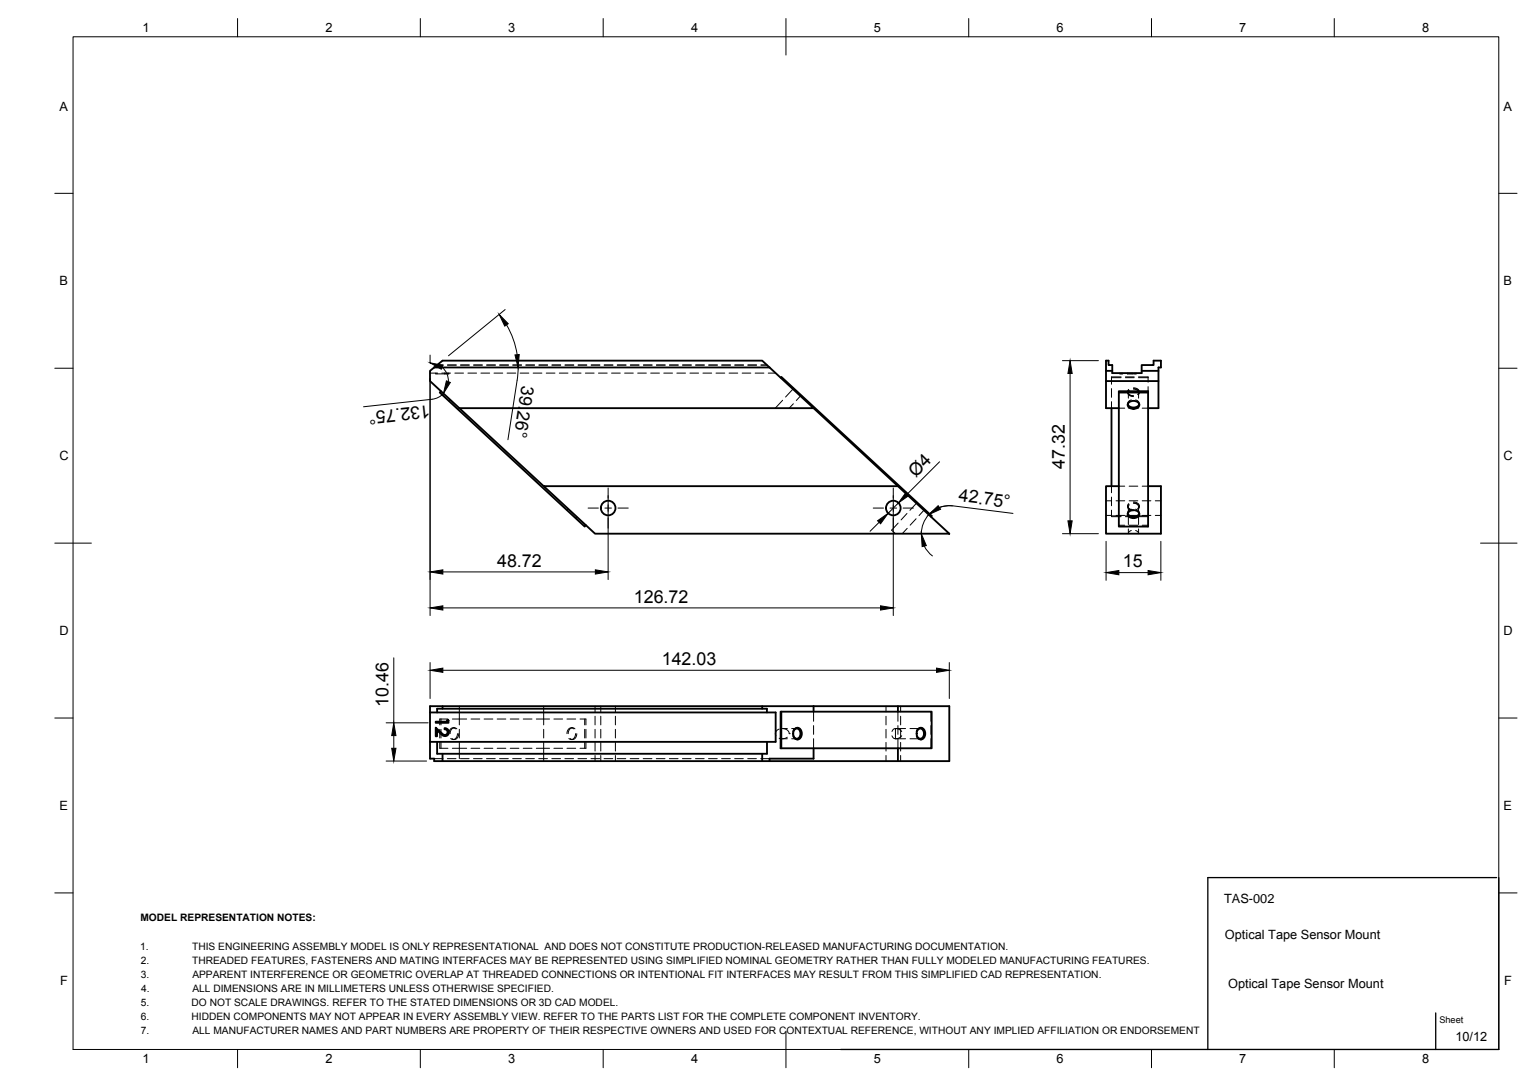
ISO-10303-21;
HEADER;
/* Generated by software containing ST-Developer
 * from STEP Tools, Inc. (www.steptools.com) 
 */

FILE_DESCRIPTION(
/* description */ ('STEP AP214'),
/* implementation_level */ '2;1');

FILE_NAME(
/* name */ 'Optical Tape Sensor Mount.step',
/* time_stamp */ '2026-11-04T19:38:14-08:00',
/* author */ (''),
/* organization */ (''),
/* preprocessor_version */ 'ST-DEVELOPER v20.2',
/* originating_system */ 'Autodesk Translation Framework v15.17.0.0',
/* authorisation */ '');

FILE_SCHEMA (('AUTOMOTIVE_DESIGN { 1 0 10303 214 3 1 1 }'));
ENDSEC;

DATA;
#10=MECHANICAL_DESIGN_GEOMETRIC_PRESENTATION_REPRESENTATION('',(#477),#36668);
#53=B_SPLINE_SURFACE_WITH_KNOTS('',3,1,((#33152,#33153),(#33154,#33155),
(#33156,#33157),(#33158,#33159),(#33160,#33161),(#33162,#33163),(#33164,
#33165),(#33166,#33167),(#33168,#33169),(#33170,#33171),(#33172,#33173),
(#33174,#33175),(#33176,#33177),(#33178,#33179),(#33180,#33181),(#33182,
#33183),(#33184,#33185),(#33186,#33187),(#33188,#33189)),.UNSPECIFIED.,
 .F.,.F.,.F.,(4,1,1,1,1,1,1,1,1,1,1,1,1,1,1,1,4),(2,2),(0.,0.0619654006870562,
0.122121905638296,0.180988496849837,0.239933216451894,0.299905831106524,
0.359988847476984,0.421775741741642,0.486575826421121,0.551534804619736,
0.615017542759975,0.677258616661654,0.739729962362713,0.803050102662949,
0.866495132015699,0.931973474177149,1.),(0.,0.0239999999999995),
 .UNSPECIFIED.);
#54=B_SPLINE_SURFACE_WITH_KNOTS('',3,1,((#33213,#33214),(#33215,#33216),
(#33217,#33218),(#33219,#33220),(#33221,#33222),(#33223,#33224),(#33225,
#33226),(#33227,#33228),(#33229,#33230),(#33231,#33232),(#33233,#33234),
(#33235,#33236),(#33237,#33238),(#33239,#33240),(#33241,#33242)),
 .UNSPECIFIED.,.F.,.F.,.F.,(4,1,1,1,1,1,1,1,1,1,1,1,4),(2,2),(0.,0.110802643801324,
0.212829202347773,0.306101309823115,0.390647321116006,0.46692446936085,
0.534481039284033,0.593586940965671,0.644557004508714,0.736200452629367,
0.825024025618864,0.911985584829753,1.),(0.,0.0239999999999995),
 .UNSPECIFIED.);
#55=B_SPLINE_SURFACE_WITH_KNOTS('',3,1,((#33280,#33281),(#33282,#33283),
(#33284,#33285),(#33286,#33287),(#33288,#33289),(#33290,#33291),(#33292,
#33293),(#33294,#33295),(#33296,#33297),(#33298,#33299),(#33300,#33301),
(#33302,#33303),(#33304,#33305),(#33306,#33307),(#33308,#33309)),
 .UNSPECIFIED.,.F.,.F.,.F.,(4,1,1,1,1,1,1,1,1,1,1,1,4),(2,2),(0.,0.0987013748863702,
0.195670680385855,0.292419992908961,0.391339286967469,0.444458741764931,
0.504224579154748,0.570347591406357,0.642913825979479,0.722289816523959,
0.807922721202247,0.900470366297794,1.),(0.,0.0239999999999995),
 .UNSPECIFIED.);
#56=B_SPLINE_SURFACE_WITH_KNOTS('',3,1,((#33327,#33328),(#33329,#33330),
(#33331,#33332),(#33333,#33334),(#33335,#33336),(#33337,#33338),(#33339,
#33340),(#33341,#33342),(#33343,#33344),(#33345,#33346),(#33347,#33348),
(#33349,#33350),(#33351,#33352),(#33353,#33354),(#33355,#33356),(#33357,
#33358),(#33359,#33360),(#33361,#33362),(#33363,#33364)),.UNSPECIFIED.,
 .F.,.F.,.F.,(4,1,1,1,1,1,1,1,1,1,1,1,1,1,1,1,4),(2,2),(0.,0.0694796363669832,
0.136525003539142,0.200800892873422,0.263983206913328,0.325711144761188,
0.38727051407573,0.449492780531563,0.51295519576285,0.576266397070109,0.637574966831173,
0.697901098424494,0.757558279411561,0.81658750436506,0.876645756608308,
0.937285872938128,1.),(0.,0.0240000000000054),.UNSPECIFIED.);
#57=B_SPLINE_SURFACE_WITH_KNOTS('',3,1,((#33386,#33387),(#33388,#33389),
(#33390,#33391),(#33392,#33393),(#33394,#33395),(#33396,#33397),(#33398,
#33399),(#33400,#33401),(#33402,#33403),(#33404,#33405),(#33406,#33407),
(#33408,#33409),(#33410,#33411),(#33412,#33413),(#33414,#33415),(#33416,
#33417),(#33418,#33419),(#33420,#33421),(#33422,#33423)),.UNSPECIFIED.,
 .F.,.F.,.F.,(4,1,1,1,1,1,1,1,1,1,1,1,1,1,1,1,4),(2,2),(0.,0.0687907943906199,
0.135103289431132,0.198978674310652,0.261904299780862,0.323494969367974,
0.385195377966055,0.446969238740777,0.509764776703136,0.572250568847369,
0.633405175661155,0.693251162921754,0.752583162785671,0.812579266153423,
0.873275084920192,0.93554994289503,1.),(0.,0.0239999999999995),
 .UNSPECIFIED.);
#58=B_SPLINE_SURFACE_WITH_KNOTS('',3,1,((#33449,#33450),(#33451,#33452),
(#33453,#33454),(#33455,#33456),(#33457,#33458),(#33459,#33460),(#33461,
#33462),(#33463,#33464),(#33465,#33466),(#33467,#33468),(#33469,#33470),
(#33471,#33472),(#33473,#33474),(#33475,#33476),(#33477,#33478),(#33479,
#33480),(#33481,#33482),(#33483,#33484),(#33485,#33486)),.UNSPECIFIED.,
 .F.,.F.,.F.,(4,1,1,1,1,1,1,1,1,1,1,1,1,1,1,1,4),(2,2),(0.,0.064429890715421,
0.126529667073554,0.186743666835525,0.245897683478137,0.304053106820992,
0.362195516217047,0.420654638852463,0.480330856318868,0.540662876085596,
0.600743511343268,0.661981856833518,0.724480055372708,0.789067141037209,
0.856333336778513,0.926362064011592,1.),(0.,0.0239999999999995),
 .UNSPECIFIED.);
#345=B_SPLINE_CURVE_WITH_KNOTS('',3,(#33030,#33031,#33032,#33033,#33034,
#33035,#33036,#33037,#33038,#33039,#33040,#33041,#33042,#33043,#33044,#33045,
#33046,#33047,#33048),.UNSPECIFIED.,.F.,.F.,(4,1,1,1,1,1,1,1,1,1,1,1,1,
1,1,1,4),(0.,0.064429890715421,0.126529667073554,0.186743666835525,0.245897683478137,
0.304053106820992,0.362195516217047,0.420654638852463,0.480330856318868,
0.540662876085596,0.600743511343268,0.661981856833518,0.724480055372708,
0.789067141037209,0.856333336778513,0.926362064011592,1.),.UNSPECIFIED.);
#346=B_SPLINE_CURVE_WITH_KNOTS('',3,(#33050,#33051,#33052,#33053,#33054,
#33055,#33056,#33057,#33058,#33059,#33060,#33061,#33062,#33063,#33064,#33065,
#33066,#33067,#33068),.UNSPECIFIED.,.F.,.F.,(4,1,1,1,1,1,1,1,1,1,1,1,1,
1,1,1,4),(0.,0.0619654006870562,0.122121905638296,0.180988496849837,0.239933216451894,
0.299905831106524,0.359988847476984,0.421775741741642,0.486575826421121,
0.551534804619736,0.615017542759975,0.677258616661654,0.739729962362713,
0.803050102662949,0.866495132015699,0.931973474177149,1.),.UNSPECIFIED.);
#347=B_SPLINE_CURVE_WITH_KNOTS('',3,(#33070,#33071,#33072,#33073,#33074,
#33075,#33076,#33077,#33078,#33079,#33080,#33081,#33082,#33083,#33084),
 .UNSPECIFIED.,.F.,.F.,(4,1,1,1,1,1,1,1,1,1,1,1,4),(0.,0.110802643801324,
0.212829202347773,0.306101309823115,0.390647321116006,0.46692446936085,
0.534481039284033,0.593586940965671,0.644557004508714,0.736200452629367,
0.825024025618864,0.911985584829753,1.),.UNSPECIFIED.);
#348=B_SPLINE_CURVE_WITH_KNOTS('',3,(#33096,#33097,#33098,#33099,#33100,
#33101,#33102,#33103,#33104,#33105,#33106,#33107,#33108,#33109,#33110),
 .UNSPECIFIED.,.F.,.F.,(4,1,1,1,1,1,1,1,1,1,1,1,4),(0.,0.0987013748863702,
0.195670680385855,0.292419992908961,0.391339286967469,0.444458741764931,
0.504224579154748,0.570347591406357,0.642913825979479,0.722289816523959,
0.807922721202247,0.900470366297794,1.),.UNSPECIFIED.);
#349=B_SPLINE_CURVE_WITH_KNOTS('',3,(#33112,#33113,#33114,#33115,#33116,
#33117,#33118,#33119,#33120,#33121,#33122,#33123,#33124,#33125,#33126,#33127,
#33128,#33129,#33130),.UNSPECIFIED.,.F.,.F.,(4,1,1,1,1,1,1,1,1,1,1,1,1,
1,1,1,4),(0.,0.0694796363669832,0.136525003539142,0.200800892873422,0.263983206913328,
0.325711144761188,0.38727051407573,0.449492780531563,0.51295519576285,0.576266397070109,
0.637574966831173,0.697901098424494,0.757558279411561,0.81658750436506,
0.876645756608308,0.937285872938128,1.),.UNSPECIFIED.);
#350=B_SPLINE_CURVE_WITH_KNOTS('',3,(#33132,#33133,#33134,#33135,#33136,
#33137,#33138,#33139,#33140,#33141,#33142,#33143,#33144,#33145,#33146,#33147,
#33148,#33149,#33150),.UNSPECIFIED.,.F.,.F.,(4,1,1,1,1,1,1,1,1,1,1,1,1,
1,1,1,4),(0.,0.0687907943906199,0.135103289431132,0.198978674310652,0.261904299780862,
0.323494969367974,0.385195377966055,0.446969238740777,0.509764776703136,
0.572250568847369,0.633405175661155,0.693251162921754,0.752583162785671,
0.812579266153423,0.873275084920192,0.93554994289503,1.),.UNSPECIFIED.);
#351=B_SPLINE_CURVE_WITH_KNOTS('',3,(#33192,#33193,#33194,#33195,#33196,
#33197,#33198,#33199,#33200,#33201,#33202,#33203,#33204,#33205,#33206,#33207,
#33208,#33209,#33210),.UNSPECIFIED.,.F.,.F.,(4,1,1,1,1,1,1,1,1,1,1,1,1,
1,1,1,4),(0.,0.0619654006870562,0.122121905638296,0.180988496849837,0.239933216451894,
0.299905831106524,0.359988847476984,0.421775741741642,0.486575826421121,
0.551534804619736,0.615017542759975,0.677258616661654,0.739729962362713,
0.803050102662949,0.866495132015699,0.931973474177149,1.),.UNSPECIFIED.);
#352=B_SPLINE_CURVE_WITH_KNOTS('',3,(#33244,#33245,#33246,#33247,#33248,
#33249,#33250,#33251,#33252,#33253,#33254,#33255,#33256,#33257,#33258),
 .UNSPECIFIED.,.F.,.F.,(4,1,1,1,1,1,1,1,1,1,1,1,4),(0.,0.110802643801324,
0.212829202347773,0.306101309823115,0.390647321116006,0.46692446936085,
0.534481039284033,0.593586940965671,0.644557004508714,0.736200452629367,
0.825024025618864,0.911985584829753,1.),.UNSPECIFIED.);
#353=B_SPLINE_CURVE_WITH_KNOTS('',3,(#33311,#33312,#33313,#33314,#33315,
#33316,#33317,#33318,#33319,#33320,#33321,#33322,#33323,#33324,#33325),
 .UNSPECIFIED.,.F.,.F.,(4,1,1,1,1,1,1,1,1,1,1,1,4),(0.,0.0987013748863702,
0.195670680385855,0.292419992908961,0.391339286967469,0.444458741764931,
0.504224579154748,0.570347591406357,0.642913825979479,0.722289816523959,
0.807922721202247,0.900470366297794,1.),.UNSPECIFIED.);
#354=B_SPLINE_CURVE_WITH_KNOTS('',3,(#33366,#33367,#33368,#33369,#33370,
#33371,#33372,#33373,#33374,#33375,#33376,#33377,#33378,#33379,#33380,#33381,
#33382,#33383,#33384),.UNSPECIFIED.,.F.,.F.,(4,1,1,1,1,1,1,1,1,1,1,1,1,
1,1,1,4),(0.,0.0694796363669832,0.136525003539142,0.200800892873422,0.263983206913328,
0.325711144761188,0.38727051407573,0.449492780531563,0.51295519576285,0.576266397070109,
0.637574966831173,0.697901098424494,0.757558279411561,0.81658750436506,
0.876645756608308,0.937285872938128,1.),.UNSPECIFIED.);
#355=B_SPLINE_CURVE_WITH_KNOTS('',3,(#33425,#33426,#33427,#33428,#33429,
#33430,#33431,#33432,#33433,#33434,#33435,#33436,#33437,#33438,#33439,#33440,
#33441,#33442,#33443),.UNSPECIFIED.,.F.,.F.,(4,1,1,1,1,1,1,1,1,1,1,1,1,
1,1,1,4),(0.,0.0687907943906199,0.135103289431132,0.198978674310652,0.261904299780862,
0.323494969367974,0.385195377966055,0.446969238740777,0.509764776703136,
0.572250568847369,0.633405175661155,0.693251162921754,0.752583162785671,
0.812579266153423,0.873275084920192,0.93554994289503,1.),.UNSPECIFIED.);
#356=B_SPLINE_CURVE_WITH_KNOTS('',3,(#33487,#33488,#33489,#33490,#33491,
#33492,#33493,#33494,#33495,#33496,#33497,#33498,#33499,#33500,#33501,#33502,
#33503,#33504,#33505),.UNSPECIFIED.,.F.,.F.,(4,1,1,1,1,1,1,1,1,1,1,1,1,
1,1,1,4),(0.,0.064429890715421,0.126529667073554,0.186743666835525,0.245897683478137,
0.304053106820992,0.362195516217047,0.420654638852463,0.480330856318868,
0.540662876085596,0.600743511343268,0.661981856833518,0.724480055372708,
0.789067141037209,0.856333336778513,0.926362064011592,1.),.UNSPECIFIED.);
#430=ELLIPSE('',#19087,1.9066404831829,1.40000000000002);
#431=ELLIPSE('',#19093,1.9066404831826,1.40000000000005);
#457=SHAPE_REPRESENTATION_RELATIONSHIP('SRR','None',#36713,#467);
#467=ADVANCED_BREP_SHAPE_REPRESENTATION('',(#487),#36665);
#477=STYLED_ITEM('',(#36769),#487);
#487=MANIFOLD_SOLID_BREP('Body1',#17800);
#702=CYLINDRICAL_SURFACE('',#19086,1.4);
#703=CYLINDRICAL_SURFACE('',#19092,1.4);
#704=CYLINDRICAL_SURFACE('',#19121,1.6);
#705=CYLINDRICAL_SURFACE('',#19123,1.6);
#706=CYLINDRICAL_SURFACE('',#19138,2.);
#707=CYLINDRICAL_SURFACE('',#19139,2.);
#708=CYLINDRICAL_SURFACE('',#19147,1.6);
#709=CYLINDRICAL_SURFACE('',#19149,1.6);
#942=FACE_BOUND('',#3354,.T.);
#943=FACE_BOUND('',#3355,.T.);
#944=FACE_BOUND('',#3358,.T.);
#945=FACE_BOUND('',#3359,.T.);
#946=FACE_BOUND('',#3361,.T.);
#947=FACE_BOUND('',#3362,.T.);
#948=FACE_BOUND('',#3367,.T.);
#949=FACE_BOUND('',#3371,.T.);
#950=FACE_BOUND('',#3373,.T.);
#951=FACE_BOUND('',#3381,.T.);
#952=FACE_BOUND('',#3382,.T.);
#953=FACE_BOUND('',#3387,.T.);
#954=FACE_BOUND('',#3396,.T.);
#955=FACE_BOUND('',#3397,.T.);
#1440=CIRCLE('',#19088,1.4);
#1441=CIRCLE('',#19090,1.4);
#1442=CIRCLE('',#19091,1.4);
#1443=CIRCLE('',#19094,1.4);
#1444=CIRCLE('',#19118,1.6);
#1445=CIRCLE('',#19120,1.6);
#1446=CIRCLE('',#19122,1.6);
#1447=CIRCLE('',#19124,1.6);
#1448=CIRCLE('',#19132,2.);
#1449=CIRCLE('',#19133,2.);
#1450=CIRCLE('',#19135,2.);
#1451=CIRCLE('',#19136,2.);
#1452=CIRCLE('',#19144,1.6);
#1453=CIRCLE('',#19146,1.6);
#1454=CIRCLE('',#19148,1.6);
#1455=CIRCLE('',#19150,1.6);
#2217=FACE_OUTER_BOUND('',#3314,.T.);
#2218=FACE_OUTER_BOUND('',#3315,.T.);
#2219=FACE_OUTER_BOUND('',#3316,.T.);
#2220=FACE_OUTER_BOUND('',#3317,.T.);
#2221=FACE_OUTER_BOUND('',#3318,.T.);
#2222=FACE_OUTER_BOUND('',#3319,.T.);
#2223=FACE_OUTER_BOUND('',#3320,.T.);
#2224=FACE_OUTER_BOUND('',#3321,.T.);
#2225=FACE_OUTER_BOUND('',#3322,.T.);
#2226=FACE_OUTER_BOUND('',#3323,.T.);
#2227=FACE_OUTER_BOUND('',#3324,.T.);
#2228=FACE_OUTER_BOUND('',#3325,.T.);
#2229=FACE_OUTER_BOUND('',#3326,.T.);
#2230=FACE_OUTER_BOUND('',#3327,.T.);
#2231=FACE_OUTER_BOUND('',#3328,.T.);
#2232=FACE_OUTER_BOUND('',#3329,.T.);
#2233=FACE_OUTER_BOUND('',#3330,.T.);
#2234=FACE_OUTER_BOUND('',#3331,.T.);
#2235=FACE_OUTER_BOUND('',#3332,.T.);
#2236=FACE_OUTER_BOUND('',#3333,.T.);
#2237=FACE_OUTER_BOUND('',#3334,.T.);
#2238=FACE_OUTER_BOUND('',#3335,.T.);
#2239=FACE_OUTER_BOUND('',#3336,.T.);
#2240=FACE_OUTER_BOUND('',#3337,.T.);
#2241=FACE_OUTER_BOUND('',#3338,.T.);
#2242=FACE_OUTER_BOUND('',#3339,.T.);
#2243=FACE_OUTER_BOUND('',#3340,.T.);
#2244=FACE_OUTER_BOUND('',#3341,.T.);
#2245=FACE_OUTER_BOUND('',#3342,.T.);
#2246=FACE_OUTER_BOUND('',#3343,.T.);
#2247=FACE_OUTER_BOUND('',#3344,.T.);
#2248=FACE_OUTER_BOUND('',#3345,.T.);
#2249=FACE_OUTER_BOUND('',#3346,.T.);
#2250=FACE_OUTER_BOUND('',#3347,.T.);
#2251=FACE_OUTER_BOUND('',#3348,.T.);
#2252=FACE_OUTER_BOUND('',#3349,.T.);
#2253=FACE_OUTER_BOUND('',#3350,.T.);
#2254=FACE_OUTER_BOUND('',#3351,.T.);
#2255=FACE_OUTER_BOUND('',#3352,.T.);
#2256=FACE_OUTER_BOUND('',#3353,.T.);
#2257=FACE_OUTER_BOUND('',#3356,.T.);
#2258=FACE_OUTER_BOUND('',#3357,.T.);
#2259=FACE_OUTER_BOUND('',#3360,.T.);
#2260=FACE_OUTER_BOUND('',#3363,.T.);
#2261=FACE_OUTER_BOUND('',#3364,.T.);
#2262=FACE_OUTER_BOUND('',#3365,.T.);
#2263=FACE_OUTER_BOUND('',#3366,.T.);
#2264=FACE_OUTER_BOUND('',#3368,.T.);
#2265=FACE_OUTER_BOUND('',#3369,.T.);
#2266=FACE_OUTER_BOUND('',#3370,.T.);
#2267=FACE_OUTER_BOUND('',#3372,.T.);
#2268=FACE_OUTER_BOUND('',#3374,.T.);
#2269=FACE_OUTER_BOUND('',#3375,.T.);
#2270=FACE_OUTER_BOUND('',#3376,.T.);
#2271=FACE_OUTER_BOUND('',#3377,.T.);
#2272=FACE_OUTER_BOUND('',#3378,.T.);
#2273=FACE_OUTER_BOUND('',#3379,.T.);
#2274=FACE_OUTER_BOUND('',#3380,.T.);
#2275=FACE_OUTER_BOUND('',#3383,.T.);
#2276=FACE_OUTER_BOUND('',#3384,.T.);
#2277=FACE_OUTER_BOUND('',#3385,.T.);
#2278=FACE_OUTER_BOUND('',#3386,.T.);
#2279=FACE_OUTER_BOUND('',#3388,.T.);
#2280=FACE_OUTER_BOUND('',#3389,.T.);
#2281=FACE_OUTER_BOUND('',#3390,.T.);
#2282=FACE_OUTER_BOUND('',#3391,.T.);
#2283=FACE_OUTER_BOUND('',#3392,.T.);
#2284=FACE_OUTER_BOUND('',#3393,.T.);
#2285=FACE_OUTER_BOUND('',#3394,.T.);
#2286=FACE_OUTER_BOUND('',#3395,.T.);
#3314=EDGE_LOOP('',(#15064,#15065,#15066,#15067));
#3315=EDGE_LOOP('',(#15068,#15069,#15070));
#3316=EDGE_LOOP('',(#15071,#15072,#15073,#15074,#15075,#15076));
#3317=EDGE_LOOP('',(#15077,#15078,#15079,#15080,#15081,#15082));
#3318=EDGE_LOOP('',(#15083,#15084,#15085,#15086));
#3319=EDGE_LOOP('',(#15087,#15088,#15089,#15090));
#3320=EDGE_LOOP('',(#15091,#15092,#15093,#15094));
#3321=EDGE_LOOP('',(#15095,#15096,#15097,#15098));
#3322=EDGE_LOOP('',(#15099,#15100,#15101,#15102));
#3323=EDGE_LOOP('',(#15103,#15104,#15105,#15106));
#3324=EDGE_LOOP('',(#15107,#15108,#15109,#15110,#15111,#15112,#15113,#15114,
#15115,#15116,#15117,#15118));
#3325=EDGE_LOOP('',(#15119,#15120,#15121,#15122));
#3326=EDGE_LOOP('',(#15123,#15124,#15125,#15126));
#3327=EDGE_LOOP('',(#15127,#15128,#15129,#15130));
#3328=EDGE_LOOP('',(#15131,#15132,#15133,#15134));
#3329=EDGE_LOOP('',(#15135,#15136,#15137,#15138));
#3330=EDGE_LOOP('',(#15139,#15140,#15141,#15142));
#3331=EDGE_LOOP('',(#15143,#15144,#15145,#15146));
#3332=EDGE_LOOP('',(#15147,#15148,#15149,#15150));
#3333=EDGE_LOOP('',(#15151,#15152,#15153,#15154));
#3334=EDGE_LOOP('',(#15155,#15156,#15157,#15158));
#3335=EDGE_LOOP('',(#15159,#15160,#15161,#15162));
#3336=EDGE_LOOP('',(#15163,#15164,#15165,#15166));
#3337=EDGE_LOOP('',(#15167,#15168,#15169,#15170,#15171));
#3338=EDGE_LOOP('',(#15172,#15173,#15174,#15175));
#3339=EDGE_LOOP('',(#15176,#15177,#15178,#15179));
#3340=EDGE_LOOP('',(#15180,#15181,#15182,#15183));
#3341=EDGE_LOOP('',(#15184,#15185,#15186,#15187));
#3342=EDGE_LOOP('',(#15188,#15189,#15190,#15191,#15192));
#3343=EDGE_LOOP('',(#15193,#15194,#15195,#15196));
#3344=EDGE_LOOP('',(#15197,#15198,#15199,#15200,#15201,#15202));
#3345=EDGE_LOOP('',(#15203));
#3346=EDGE_LOOP('',(#15204));
#3347=EDGE_LOOP('',(#15205,#15206,#15207,#15208));
#3348=EDGE_LOOP('',(#15209,#15210,#15211,#15212));
#3349=EDGE_LOOP('',(#15213,#15214,#15215,#15216,#15217,#15218));
#3350=EDGE_LOOP('',(#15219,#15220,#15221,#15222));
#3351=EDGE_LOOP('',(#15223,#15224,#15225,#15226,#15227,#15228));
#3352=EDGE_LOOP('',(#15229,#15230,#15231,#15232));
#3353=EDGE_LOOP('',(#15233,#15234,#15235,#15236));
#3354=EDGE_LOOP('',(#15237));
#3355=EDGE_LOOP('',(#15238));
#3356=EDGE_LOOP('',(#15239,#15240,#15241,#15242));
#3357=EDGE_LOOP('',(#15243,#15244,#15245,#15246));
#3358=EDGE_LOOP('',(#15247));
#3359=EDGE_LOOP('',(#15248));
#3360=EDGE_LOOP('',(#15249,#15250,#15251,#15252));
#3361=EDGE_LOOP('',(#15253));
#3362=EDGE_LOOP('',(#15254));
#3363=EDGE_LOOP('',(#15255,#15256,#15257,#15258,#15259,#15260,#15261,#15262));
#3364=EDGE_LOOP('',(#15263,#15264,#15265,#15266));
#3365=EDGE_LOOP('',(#15267,#15268,#15269,#15270));
#3366=EDGE_LOOP('',(#15271,#15272,#15273,#15274));
#3367=EDGE_LOOP('',(#15275,#15276));
#3368=EDGE_LOOP('',(#15277,#15278,#15279,#15280,#15281,#15282,#15283,#15284));
#3369=EDGE_LOOP('',(#15285,#15286,#15287,#15288,#15289,#15290,#15291,#15292));
#3370=EDGE_LOOP('',(#15293));
#3371=EDGE_LOOP('',(#15294));
#3372=EDGE_LOOP('',(#15295));
#3373=EDGE_LOOP('',(#15296));
#3374=EDGE_LOOP('',(#15297,#15298,#15299,#15300));
#3375=EDGE_LOOP('',(#15301,#15302,#15303,#15304));
#3376=EDGE_LOOP('',(#15305,#15306,#15307,#15308,#15309,#15310));
#3377=EDGE_LOOP('',(#15311,#15312,#15313,#15314));
#3378=EDGE_LOOP('',(#15315,#15316,#15317,#15318,#15319,#15320));
#3379=EDGE_LOOP('',(#15321,#15322,#15323,#15324));
#3380=EDGE_LOOP('',(#15325,#15326,#15327,#15328));
#3381=EDGE_LOOP('',(#15329));
#3382=EDGE_LOOP('',(#15330));
#3383=EDGE_LOOP('',(#15331,#15332,#15333,#15334));
#3384=EDGE_LOOP('',(#15335,#15336,#15337,#15338,#15339,#15340));
#3385=EDGE_LOOP('',(#15341,#15342,#15343,#15344,#15345,#15346,#15347,#15348));
#3386=EDGE_LOOP('',(#15349,#15350,#15351,#15352,#15353,#15354,#15355,#15356));
#3387=EDGE_LOOP('',(#15357));
#3388=EDGE_LOOP('',(#15358,#15359,#15360,#15361,#15362,#15363,#15364,#15365,
#15366,#15367,#15368,#15369,#15370,#15371,#15372,#15373,#15374,#15375));
#3389=EDGE_LOOP('',(#15376,#15377,#15378,#15379));
#3390=EDGE_LOOP('',(#15380,#15381,#15382,#15383,#15384,#15385,#15386,#15387));
#3391=EDGE_LOOP('',(#15388,#15389,#15390,#15391,#15392,#15393,#15394,#15395));
#3392=EDGE_LOOP('',(#15396,#15397,#15398,#15399));
#3393=EDGE_LOOP('',(#15400,#15401,#15402,#15403));
#3394=EDGE_LOOP('',(#15404,#15405,#15406,#15407,#15408,#15409));
#3395=EDGE_LOOP('',(#15410,#15411,#15412,#15413));
#3396=EDGE_LOOP('',(#15414,#15415,#15416,#15417,#15418,#15419));
#3397=EDGE_LOOP('',(#15420,#15421,#15422,#15423,#15424,#15425,#15426,#15427,
#15428,#15429,#15430,#15431));
#4845=LINE('',#32976,#6555);
#4846=LINE('',#32981,#6556);
#4847=LINE('',#32988,#6557);
#4848=LINE('',#32993,#6558);
#4849=LINE('',#32995,#6559);
#4850=LINE('',#32997,#6560);
#4851=LINE('',#32999,#6561);
#4852=LINE('',#33001,#6562);
#4853=LINE('',#33002,#6563);
#4854=LINE('',#33006,#6564);
#4855=LINE('',#33007,#6565);
#4856=LINE('',#33008,#6566);
#4857=LINE('',#33011,#6567);
#4858=LINE('',#33012,#6568);
#4859=LINE('',#33015,#6569);
#4860=LINE('',#33016,#6570);
#4861=LINE('',#33019,#6571);
#4862=LINE('',#33020,#6572);
#4863=LINE('',#33023,#6573);
#4864=LINE('',#33024,#6574);
#4865=LINE('',#33026,#6575);
#4866=LINE('',#33086,#6576);
#4867=LINE('',#33088,#6577);
#4868=LINE('',#33090,#6578);
#4869=LINE('',#33092,#6579);
#4870=LINE('',#33094,#6580);
#4871=LINE('',#33151,#6581);
#4872=LINE('',#33211,#6582);
#4873=LINE('',#33212,#6583);
#4874=LINE('',#33259,#6584);
#4875=LINE('',#33262,#6585);
#4876=LINE('',#33263,#6586);
#4877=LINE('',#33266,#6587);
#4878=LINE('',#33267,#6588);
#4879=LINE('',#33270,#6589);
#4880=LINE('',#33271,#6590);
#4881=LINE('',#33274,#6591);
#4882=LINE('',#33275,#6592);
#4883=LINE('',#33278,#6593);
#4884=LINE('',#33279,#6594);
#4885=LINE('',#33326,#6595);
#4886=LINE('',#33385,#6596);
#4887=LINE('',#33444,#6597);
#4888=LINE('',#33447,#6598);
#4889=LINE('',#33448,#6599);
#4890=LINE('',#33509,#6600);
#4891=LINE('',#33511,#6601);
#4892=LINE('',#33513,#6602);
#4893=LINE('',#33515,#6603);
#4894=LINE('',#33516,#6604);
#4895=LINE('',#33520,#6605);
#4896=LINE('',#33521,#6606);
#4897=LINE('',#33522,#6607);
#4898=LINE('',#33526,#6608);
#4899=LINE('',#33527,#6609);
#4900=LINE('',#33528,#6610);
#4901=LINE('',#33532,#6611);
#4902=LINE('',#33534,#6612);
#4903=LINE('',#33536,#6613);
#4904=LINE('',#33537,#6614);
#4905=LINE('',#33541,#6615);
#4906=LINE('',#33542,#6616);
#4907=LINE('',#33543,#6617);
#4908=LINE('',#33547,#6618);
#4909=LINE('',#33549,#6619);
#4910=LINE('',#33550,#6620);
#4911=LINE('',#33551,#6621);
#4912=LINE('',#33555,#6622);
#4913=LINE('',#33557,#6623);
#4914=LINE('',#33559,#6624);
#4915=LINE('',#33560,#6625);
#4916=LINE('',#33564,#6626);
#4917=LINE('',#33566,#6627);
#4918=LINE('',#33568,#6628);
#4919=LINE('',#33569,#6629);
#4920=LINE('',#33570,#6630);
#4921=LINE('',#33580,#6631);
#4922=LINE('',#33584,#6632);
#4923=LINE('',#33588,#6633);
#4924=LINE('',#33590,#6634);
#4925=LINE('',#33592,#6635);
#4926=LINE('',#33594,#6636);
#4927=LINE('',#33596,#6637);
#4928=LINE('',#33597,#6638);
#4929=LINE('',#33600,#6639);
#4930=LINE('',#33602,#6640);
#4931=LINE('',#33603,#6641);
#4932=LINE('',#33607,#6642);
#4933=LINE('',#33609,#6643);
#4934=LINE('',#33610,#6644);
#4935=LINE('',#33612,#6645);
#4936=LINE('',#33613,#6646);
#4937=LINE('',#33615,#6647);
#4938=LINE('',#33616,#6648);
#4939=LINE('',#33619,#6649);
#4940=LINE('',#33620,#6650);
#4941=LINE('',#33624,#6651);
#4942=LINE('',#33626,#6652);
#4943=LINE('',#33628,#6653);
#4944=LINE('',#33629,#6654);
#4945=LINE('',#33637,#6655);
#4946=LINE('',#33639,#6656);
#4947=LINE('',#33641,#6657);
#4948=LINE('',#33642,#6658);
#4949=LINE('',#33648,#6659);
#4950=LINE('',#33649,#6660);
#4951=LINE('',#33650,#6661);
#4952=LINE('',#33652,#6662);
#4953=LINE('',#33654,#6663);
#4954=LINE('',#33656,#6664);
#4955=LINE('',#33660,#6665);
#4956=LINE('',#33662,#6666);
#4957=LINE('',#33663,#6667);
#4958=LINE('',#33665,#6668);
#4959=LINE('',#33666,#6669);
#4960=LINE('',#33668,#6670);
#4961=LINE('',#33678,#6671);
#4962=LINE('',#33682,#6672);
#4963=LINE('',#33685,#6673);
#4964=LINE('',#33687,#6674);
#4965=LINE('',#33689,#6675);
#4966=LINE('',#33691,#6676);
#4967=LINE('',#33692,#6677);
#4968=LINE('',#33695,#6678);
#4969=LINE('',#33696,#6679);
#4970=LINE('',#33700,#6680);
#4971=LINE('',#33701,#6681);
#4972=LINE('',#33703,#6682);
#4973=LINE('',#33704,#6683);
#4974=LINE('',#33706,#6684);
#4975=LINE('',#33707,#6685);
#4976=LINE('',#33711,#6686);
#4977=LINE('',#33713,#6687);
#4978=LINE('',#33714,#6688);
#4979=LINE('',#33718,#6689);
#4980=LINE('',#33720,#6690);
#4981=LINE('',#33722,#6691);
#4982=LINE('',#33724,#6692);
#4983=LINE('',#33726,#6693);
#4984=LINE('',#33727,#6694);
#4985=LINE('',#33729,#6695);
#4986=LINE('',#33730,#6696);
#4987=LINE('',#33731,#6697);
#4988=LINE('',#33733,#6698);
#4989=LINE('',#33734,#6699);
#4990=LINE('',#33735,#6700);
#4991=LINE('',#33737,#6701);
#4992=LINE('',#33738,#6702);
#4993=LINE('',#33739,#6703);
#4994=LINE('',#33741,#6704);
#4995=LINE('',#33743,#6705);
#4996=LINE('',#33745,#6706);
#4997=LINE('',#33746,#6707);
#4998=LINE('',#33749,#6708);
#6555=VECTOR('',#23043,1.4);
#6556=VECTOR('',#23048,1000.);
#6557=VECTOR('',#23057,1.4);
#6558=VECTOR('',#23062,1000.);
#6559=VECTOR('',#23063,1000.);
#6560=VECTOR('',#23064,1000.);
#6561=VECTOR('',#23065,1000.);
#6562=VECTOR('',#23066,1000.);
#6563=VECTOR('',#23067,1000.);
#6564=VECTOR('',#23070,1000.);
#6565=VECTOR('',#23071,1000.);
#6566=VECTOR('',#23072,1000.);
#6567=VECTOR('',#23075,1000.);
#6568=VECTOR('',#23076,1000.);
#6569=VECTOR('',#23079,1000.);
#6570=VECTOR('',#23080,1000.);
#6571=VECTOR('',#23083,1000.);
#6572=VECTOR('',#23084,1000.);
#6573=VECTOR('',#23087,1000.);
#6574=VECTOR('',#23088,1000.);
#6575=VECTOR('',#23091,1000.);
#6576=VECTOR('',#23094,1000.);
#6577=VECTOR('',#23095,1000.);
#6578=VECTOR('',#23096,1000.);
#6579=VECTOR('',#23097,1000.);
#6580=VECTOR('',#23098,1000.);
#6581=VECTOR('',#23099,1000.);
#6582=VECTOR('',#23100,1000.);
#6583=VECTOR('',#23101,1000.);
#6584=VECTOR('',#23102,1000.);
#6585=VECTOR('',#23105,1000.);
#6586=VECTOR('',#23106,1000.);
#6587=VECTOR('',#23109,1000.);
#6588=VECTOR('',#23110,1000.);
#6589=VECTOR('',#23113,1000.);
#6590=VECTOR('',#23114,1000.);
#6591=VECTOR('',#23117,1000.);
#6592=VECTOR('',#23118,1000.);
#6593=VECTOR('',#23121,1000.);
#6594=VECTOR('',#23122,1000.);
#6595=VECTOR('',#23123,1000.);
#6596=VECTOR('',#23124,1000.);
#6597=VECTOR('',#23125,1000.);
#6598=VECTOR('',#23128,1000.);
#6599=VECTOR('',#23129,1000.);
#6600=VECTOR('',#23132,1000.);
#6601=VECTOR('',#23133,1000.);
#6602=VECTOR('',#23134,1000.);
#6603=VECTOR('',#23135,1000.);
#6604=VECTOR('',#23136,1000.);
#6605=VECTOR('',#23139,1000.);
#6606=VECTOR('',#23140,1000.);
#6607=VECTOR('',#23141,1000.);
#6608=VECTOR('',#23144,1000.);
#6609=VECTOR('',#23145,1000.);
#6610=VECTOR('',#23146,1000.);
#6611=VECTOR('',#23149,1000.);
#6612=VECTOR('',#23150,1000.);
#6613=VECTOR('',#23151,1000.);
#6614=VECTOR('',#23152,1000.);
#6615=VECTOR('',#23155,1000.);
#6616=VECTOR('',#23156,1000.);
#6617=VECTOR('',#23157,1000.);
#6618=VECTOR('',#23160,1000.);
#6619=VECTOR('',#23161,1000.);
#6620=VECTOR('',#23162,1000.);
#6621=VECTOR('',#23163,1000.);
#6622=VECTOR('',#23166,1000.);
#6623=VECTOR('',#23167,1000.);
#6624=VECTOR('',#23168,1000.);
#6625=VECTOR('',#23169,1000.);
#6626=VECTOR('',#23172,1000.);
#6627=VECTOR('',#23173,1000.);
#6628=VECTOR('',#23174,1000.);
#6629=VECTOR('',#23175,1000.);
#6630=VECTOR('',#23176,1000.);
#6631=VECTOR('',#23189,1.6);
#6632=VECTOR('',#23194,1.6);
#6633=VECTOR('',#23197,1000.);
#6634=VECTOR('',#23198,1000.);
#6635=VECTOR('',#23199,1000.);
#6636=VECTOR('',#23200,1000.);
#6637=VECTOR('',#23201,1000.);
#6638=VECTOR('',#23202,1000.);
#6639=VECTOR('',#23205,1000.);
#6640=VECTOR('',#23206,1000.);
#6641=VECTOR('',#23207,1000.);
#6642=VECTOR('',#23210,1000.);
#6643=VECTOR('',#23211,1000.);
#6644=VECTOR('',#23212,1000.);
#6645=VECTOR('',#23213,1000.);
#6646=VECTOR('',#23214,1000.);
#6647=VECTOR('',#23217,1000.);
#6648=VECTOR('',#23218,1000.);
#6649=VECTOR('',#23223,1000.);
#6650=VECTOR('',#23224,1000.);
#6651=VECTOR('',#23227,1000.);
#6652=VECTOR('',#23228,1000.);
#6653=VECTOR('',#23229,1000.);
#6654=VECTOR('',#23230,1000.);
#6655=VECTOR('',#23237,1000.);
#6656=VECTOR('',#23238,1000.);
#6657=VECTOR('',#23239,1000.);
#6658=VECTOR('',#23240,1000.);
#6659=VECTOR('',#23247,1000.);
#6660=VECTOR('',#23248,1000.);
#6661=VECTOR('',#23249,1000.);
#6662=VECTOR('',#23252,2.);
#6663=VECTOR('',#23255,2.);
#6664=VECTOR('',#23258,1000.);
#6665=VECTOR('',#23261,1000.);
#6666=VECTOR('',#23262,1000.);
#6667=VECTOR('',#23263,1000.);
#6668=VECTOR('',#23264,1000.);
#6669=VECTOR('',#23265,1000.);
#6670=VECTOR('',#23268,1000.);
#6671=VECTOR('',#23281,1.6);
#6672=VECTOR('',#23286,1.6);
#6673=VECTOR('',#23289,1000.);
#6674=VECTOR('',#23290,1000.);
#6675=VECTOR('',#23291,1000.);
#6676=VECTOR('',#23292,1000.);
#6677=VECTOR('',#23293,1000.);
#6678=VECTOR('',#23296,1000.);
#6679=VECTOR('',#23297,1000.);
#6680=VECTOR('',#23300,1000.);
#6681=VECTOR('',#23301,1000.);
#6682=VECTOR('',#23302,1000.);
#6683=VECTOR('',#23303,1000.);
#6684=VECTOR('',#23306,1000.);
#6685=VECTOR('',#23307,1000.);
#6686=VECTOR('',#23312,1000.);
#6687=VECTOR('',#23313,1000.);
#6688=VECTOR('',#23314,1000.);
#6689=VECTOR('',#23317,1000.);
#6690=VECTOR('',#23318,1000.);
#6691=VECTOR('',#23319,1000.);
#6692=VECTOR('',#23320,1000.);
#6693=VECTOR('',#23321,1000.);
#6694=VECTOR('',#23322,1000.);
#6695=VECTOR('',#23325,1000.);
#6696=VECTOR('',#23326,1000.);
#6697=VECTOR('',#23327,1000.);
#6698=VECTOR('',#23330,1000.);
#6699=VECTOR('',#23331,1000.);
#6700=VECTOR('',#23332,1000.);
#6701=VECTOR('',#23335,1000.);
#6702=VECTOR('',#23336,1000.);
#6703=VECTOR('',#23337,1000.);
#6704=VECTOR('',#23340,1000.);
#6705=VECTOR('',#23343,1000.);
#6706=VECTOR('',#23346,1000.);
#6707=VECTOR('',#23347,1000.);
#6708=VECTOR('',#23352,1000.);
#8247=VERTEX_POINT('',#32973);
#8248=VERTEX_POINT('',#32975);
#8249=VERTEX_POINT('',#32979);
#8250=VERTEX_POINT('',#32980);
#8251=VERTEX_POINT('',#32982);
#8252=VERTEX_POINT('',#32987);
#8253=VERTEX_POINT('',#32991);
#8254=VERTEX_POINT('',#32992);
#8255=VERTEX_POINT('',#32994);
#8256=VERTEX_POINT('',#32996);
#8257=VERTEX_POINT('',#32998);
#8258=VERTEX_POINT('',#33000);
#8259=VERTEX_POINT('',#33004);
#8260=VERTEX_POINT('',#33005);
#8261=VERTEX_POINT('',#33010);
#8262=VERTEX_POINT('',#33014);
#8263=VERTEX_POINT('',#33018);
#8264=VERTEX_POINT('',#33022);
#8265=VERTEX_POINT('',#33028);
#8266=VERTEX_POINT('',#33029);
#8267=VERTEX_POINT('',#33049);
#8268=VERTEX_POINT('',#33069);
#8269=VERTEX_POINT('',#33085);
#8270=VERTEX_POINT('',#33087);
#8271=VERTEX_POINT('',#33089);
#8272=VERTEX_POINT('',#33091);
#8273=VERTEX_POINT('',#33093);
#8274=VERTEX_POINT('',#33095);
#8275=VERTEX_POINT('',#33111);
#8276=VERTEX_POINT('',#33131);
#8277=VERTEX_POINT('',#33190);
#8278=VERTEX_POINT('',#33191);
#8279=VERTEX_POINT('',#33243);
#8280=VERTEX_POINT('',#33261);
#8281=VERTEX_POINT('',#33265);
#8282=VERTEX_POINT('',#33269);
#8283=VERTEX_POINT('',#33273);
#8284=VERTEX_POINT('',#33277);
#8285=VERTEX_POINT('',#33310);
#8286=VERTEX_POINT('',#33365);
#8287=VERTEX_POINT('',#33424);
#8288=VERTEX_POINT('',#33446);
#8289=VERTEX_POINT('',#33507);
#8290=VERTEX_POINT('',#33508);
#8291=VERTEX_POINT('',#33510);
#8292=VERTEX_POINT('',#33512);
#8293=VERTEX_POINT('',#33514);
#8294=VERTEX_POINT('',#33518);
#8295=VERTEX_POINT('',#33519);
#8296=VERTEX_POINT('',#33524);
#8297=VERTEX_POINT('',#33525);
#8298=VERTEX_POINT('',#33530);
#8299=VERTEX_POINT('',#33531);
#8300=VERTEX_POINT('',#33533);
#8301=VERTEX_POINT('',#33535);
#8302=VERTEX_POINT('',#33539);
#8303=VERTEX_POINT('',#33540);
#8304=VERTEX_POINT('',#33545);
#8305=VERTEX_POINT('',#33546);
#8306=VERTEX_POINT('',#33548);
#8307=VERTEX_POINT('',#33553);
#8308=VERTEX_POINT('',#33554);
#8309=VERTEX_POINT('',#33556);
#8310=VERTEX_POINT('',#33558);
#8311=VERTEX_POINT('',#33562);
#8312=VERTEX_POINT('',#33563);
#8313=VERTEX_POINT('',#33565);
#8314=VERTEX_POINT('',#33567);
#8315=VERTEX_POINT('',#33572);
#8316=VERTEX_POINT('',#33575);
#8317=VERTEX_POINT('',#33578);
#8318=VERTEX_POINT('',#33582);
#8319=VERTEX_POINT('',#33586);
#8320=VERTEX_POINT('',#33587);
#8321=VERTEX_POINT('',#33589);
#8322=VERTEX_POINT('',#33591);
#8323=VERTEX_POINT('',#33593);
#8324=VERTEX_POINT('',#33595);
#8325=VERTEX_POINT('',#33599);
#8326=VERTEX_POINT('',#33601);
#8327=VERTEX_POINT('',#33605);
#8328=VERTEX_POINT('',#33606);
#8329=VERTEX_POINT('',#33608);
#8330=VERTEX_POINT('',#33611);
#8331=VERTEX_POINT('',#33622);
#8332=VERTEX_POINT('',#33623);
#8333=VERTEX_POINT('',#33625);
#8334=VERTEX_POINT('',#33627);
#8335=VERTEX_POINT('',#33630);
#8336=VERTEX_POINT('',#33632);
#8337=VERTEX_POINT('',#33635);
#8338=VERTEX_POINT('',#33636);
#8339=VERTEX_POINT('',#33638);
#8340=VERTEX_POINT('',#33640);
#8341=VERTEX_POINT('',#33643);
#8342=VERTEX_POINT('',#33645);
#8343=VERTEX_POINT('',#33658);
#8344=VERTEX_POINT('',#33659);
#8345=VERTEX_POINT('',#33661);
#8346=VERTEX_POINT('',#33664);
#8347=VERTEX_POINT('',#33670);
#8348=VERTEX_POINT('',#33673);
#8349=VERTEX_POINT('',#33676);
#8350=VERTEX_POINT('',#33680);
#8351=VERTEX_POINT('',#33684);
#8352=VERTEX_POINT('',#33686);
#8353=VERTEX_POINT('',#33688);
#8354=VERTEX_POINT('',#33690);
#8355=VERTEX_POINT('',#33694);
#8356=VERTEX_POINT('',#33698);
#8357=VERTEX_POINT('',#33699);
#8358=VERTEX_POINT('',#33702);
#8359=VERTEX_POINT('',#33710);
#8360=VERTEX_POINT('',#33712);
#8361=VERTEX_POINT('',#33716);
#8362=VERTEX_POINT('',#33717);
#8363=VERTEX_POINT('',#33719);
#8364=VERTEX_POINT('',#33721);
#8365=VERTEX_POINT('',#33723);
#8366=VERTEX_POINT('',#33725);
#10584=EDGE_CURVE('',#8247,#8247,#430,.T.);
#10585=EDGE_CURVE('',#8247,#8248,#4845,.T.);
#10586=EDGE_CURVE('',#8248,#8248,#1440,.T.);
#10587=EDGE_CURVE('',#8249,#8250,#4846,.T.);
#10588=EDGE_CURVE('',#8250,#8251,#1441,.T.);
#10589=EDGE_CURVE('',#8251,#8249,#1442,.T.);
#10590=EDGE_CURVE('',#8249,#8250,#431,.T.);
#10591=EDGE_CURVE('',#8251,#8252,#4847,.T.);
#10592=EDGE_CURVE('',#8252,#8252,#1443,.T.);
#10593=EDGE_CURVE('',#8253,#8254,#4848,.T.);
#10594=EDGE_CURVE('',#8255,#8253,#4849,.T.);
#10595=EDGE_CURVE('',#8256,#8255,#4850,.T.);
#10596=EDGE_CURVE('',#8257,#8256,#4851,.T.);
#10597=EDGE_CURVE('',#8258,#8257,#4852,.T.);
#10598=EDGE_CURVE('',#8254,#8258,#4853,.T.);
#10599=EDGE_CURVE('',#8259,#8260,#4854,.T.);
#10600=EDGE_CURVE('',#8255,#8259,#4855,.T.);
#10601=EDGE_CURVE('',#8253,#8260,#4856,.T.);
#10602=EDGE_CURVE('',#8261,#8259,#4857,.T.);
#10603=EDGE_CURVE('',#8256,#8261,#4858,.T.);
#10604=EDGE_CURVE('',#8262,#8261,#4859,.T.);
#10605=EDGE_CURVE('',#8257,#8262,#4860,.T.);
#10606=EDGE_CURVE('',#8263,#8262,#4861,.T.);
#10607=EDGE_CURVE('',#8258,#8263,#4862,.T.);
#10608=EDGE_CURVE('',#8264,#8263,#4863,.T.);
#10609=EDGE_CURVE('',#8254,#8264,#4864,.T.);
#10610=EDGE_CURVE('',#8260,#8264,#4865,.T.);
#10611=EDGE_CURVE('',#8265,#8266,#345,.T.);
#10612=EDGE_CURVE('',#8267,#8265,#346,.T.);
#10613=EDGE_CURVE('',#8268,#8267,#347,.T.);
#10614=EDGE_CURVE('',#8269,#8268,#4866,.T.);
#10615=EDGE_CURVE('',#8270,#8269,#4867,.T.);
#10616=EDGE_CURVE('',#8271,#8270,#4868,.T.);
#10617=EDGE_CURVE('',#8272,#8271,#4869,.T.);
#10618=EDGE_CURVE('',#8273,#8272,#4870,.T.);
#10619=EDGE_CURVE('',#8274,#8273,#348,.T.);
#10620=EDGE_CURVE('',#8275,#8274,#349,.T.);
#10621=EDGE_CURVE('',#8276,#8275,#350,.T.);
#10622=EDGE_CURVE('',#8266,#8276,#4871,.T.);
#10623=EDGE_CURVE('',#8277,#8278,#351,.T.);
#10624=EDGE_CURVE('',#8267,#8277,#4872,.T.);
#10625=EDGE_CURVE('',#8265,#8278,#4873,.T.);
#10626=EDGE_CURVE('',#8279,#8277,#352,.T.);
#10627=EDGE_CURVE('',#8268,#8279,#4874,.T.);
#10628=EDGE_CURVE('',#8280,#8279,#4875,.T.);
#10629=EDGE_CURVE('',#8269,#8280,#4876,.T.);
#10630=EDGE_CURVE('',#8281,#8280,#4877,.T.);
#10631=EDGE_CURVE('',#8270,#8281,#4878,.T.);
#10632=EDGE_CURVE('',#8282,#8281,#4879,.T.);
#10633=EDGE_CURVE('',#8271,#8282,#4880,.T.);
#10634=EDGE_CURVE('',#8283,#8282,#4881,.T.);
#10635=EDGE_CURVE('',#8272,#8283,#4882,.T.);
#10636=EDGE_CURVE('',#8284,#8283,#4883,.T.);
#10637=EDGE_CURVE('',#8273,#8284,#4884,.T.);
#10638=EDGE_CURVE('',#8285,#8284,#353,.T.);
#10639=EDGE_CURVE('',#8274,#8285,#4885,.T.);
#10640=EDGE_CURVE('',#8286,#8285,#354,.T.);
#10641=EDGE_CURVE('',#8275,#8286,#4886,.T.);
#10642=EDGE_CURVE('',#8287,#8286,#355,.T.);
#10643=EDGE_CURVE('',#8276,#8287,#4887,.T.);
#10644=EDGE_CURVE('',#8288,#8287,#4888,.T.);
#10645=EDGE_CURVE('',#8266,#8288,#4889,.T.);
#10646=EDGE_CURVE('',#8278,#8288,#356,.T.);
#10647=EDGE_CURVE('',#8289,#8290,#4890,.T.);
#10648=EDGE_CURVE('',#8291,#8289,#4891,.T.);
#10649=EDGE_CURVE('',#8291,#8292,#4892,.T.);
#10650=EDGE_CURVE('',#8292,#8293,#4893,.T.);
#10651=EDGE_CURVE('',#8290,#8293,#4894,.T.);
#10652=EDGE_CURVE('',#8294,#8295,#4895,.T.);
#10653=EDGE_CURVE('',#8289,#8294,#4896,.T.);
#10654=EDGE_CURVE('',#8295,#8290,#4897,.T.);
#10655=EDGE_CURVE('',#8296,#8297,#4898,.T.);
#10656=EDGE_CURVE('',#8294,#8296,#4899,.T.);
#10657=EDGE_CURVE('',#8297,#8295,#4900,.T.);
#10658=EDGE_CURVE('',#8298,#8299,#4901,.T.);
#10659=EDGE_CURVE('',#8300,#8298,#4902,.T.);
#10660=EDGE_CURVE('',#8300,#8301,#4903,.T.);
#10661=EDGE_CURVE('',#8299,#8301,#4904,.T.);
#10662=EDGE_CURVE('',#8302,#8303,#4905,.T.);
#10663=EDGE_CURVE('',#8298,#8302,#4906,.T.);
#10664=EDGE_CURVE('',#8303,#8299,#4907,.T.);
#10665=EDGE_CURVE('',#8304,#8305,#4908,.T.);
#10666=EDGE_CURVE('',#8306,#8305,#4909,.T.);
#10667=EDGE_CURVE('',#8302,#8306,#4910,.T.);
#10668=EDGE_CURVE('',#8304,#8303,#4911,.T.);
#10669=EDGE_CURVE('',#8307,#8308,#4912,.T.);
#10670=EDGE_CURVE('',#8309,#8307,#4913,.T.);
#10671=EDGE_CURVE('',#8310,#8309,#4914,.T.);
#10672=EDGE_CURVE('',#8308,#8310,#4915,.T.);
#10673=EDGE_CURVE('',#8311,#8312,#4916,.T.);
#10674=EDGE_CURVE('',#8313,#8312,#4917,.T.);
#10675=EDGE_CURVE('',#8314,#8313,#4918,.T.);
#10676=EDGE_CURVE('',#8307,#8314,#4919,.T.);
#10677=EDGE_CURVE('',#8311,#8308,#4920,.T.);
#10678=EDGE_CURVE('',#8315,#8315,#1444,.T.);
#10679=EDGE_CURVE('',#8316,#8316,#1445,.T.);
#10680=EDGE_CURVE('',#8317,#8317,#1446,.T.);
#10681=EDGE_CURVE('',#8317,#8315,#4921,.T.);
#10682=EDGE_CURVE('',#8318,#8318,#1447,.T.);
#10683=EDGE_CURVE('',#8318,#8316,#4922,.T.);
#10684=EDGE_CURVE('',#8319,#8320,#4923,.T.);
#10685=EDGE_CURVE('',#8320,#8321,#4924,.T.);
#10686=EDGE_CURVE('',#8321,#8322,#4925,.T.);
#10687=EDGE_CURVE('',#8323,#8322,#4926,.T.);
#10688=EDGE_CURVE('',#8324,#8323,#4927,.T.);
#10689=EDGE_CURVE('',#8324,#8319,#4928,.T.);
#10690=EDGE_CURVE('',#8325,#8319,#4929,.T.);
#10691=EDGE_CURVE('',#8326,#8324,#4930,.T.);
#10692=EDGE_CURVE('',#8326,#8325,#4931,.T.);
#10693=EDGE_CURVE('',#8327,#8328,#4932,.T.);
#10694=EDGE_CURVE('',#8328,#8329,#4933,.T.);
#10695=EDGE_CURVE('',#8329,#8325,#4934,.T.);
#10696=EDGE_CURVE('',#8330,#8326,#4935,.T.);
#10697=EDGE_CURVE('',#8330,#8327,#4936,.T.);
#10698=EDGE_CURVE('',#8322,#8327,#4937,.T.);
#10699=EDGE_CURVE('',#8323,#8330,#4938,.T.);
#10700=EDGE_CURVE('',#8321,#8328,#4939,.T.);
#10701=EDGE_CURVE('',#8329,#8320,#4940,.T.);
#10702=EDGE_CURVE('',#8331,#8332,#4941,.T.);
#10703=EDGE_CURVE('',#8333,#8331,#4942,.T.);
#10704=EDGE_CURVE('',#8334,#8333,#4943,.T.);
#10705=EDGE_CURVE('',#8332,#8334,#4944,.T.);
#10706=EDGE_CURVE('',#8335,#8335,#1448,.T.);
#10707=EDGE_CURVE('',#8336,#8336,#1449,.T.);
#10708=EDGE_CURVE('',#8337,#8338,#4945,.T.);
#10709=EDGE_CURVE('',#8338,#8339,#4946,.T.);
#10710=EDGE_CURVE('',#8339,#8340,#4947,.T.);
#10711=EDGE_CURVE('',#8340,#8337,#4948,.T.);
#10712=EDGE_CURVE('',#8341,#8341,#1450,.T.);
#10713=EDGE_CURVE('',#8342,#8342,#1451,.T.);
#10714=EDGE_CURVE('',#8337,#8329,#4949,.T.);
#10715=EDGE_CURVE('',#8340,#8333,#4950,.T.);
#10716=EDGE_CURVE('',#8320,#8331,#4951,.T.);
#10717=EDGE_CURVE('',#8342,#8336,#4952,.T.);
#10718=EDGE_CURVE('',#8341,#8335,#4953,.T.);
#10719=EDGE_CURVE('',#8339,#8334,#4954,.T.);
#10720=EDGE_CURVE('',#8343,#8344,#4955,.T.);
#10721=EDGE_CURVE('',#8343,#8345,#4956,.T.);
#10722=EDGE_CURVE('',#8345,#8332,#4957,.T.);
#10723=EDGE_CURVE('',#8338,#8346,#4958,.T.);
#10724=EDGE_CURVE('',#8344,#8346,#4959,.T.);
#10725=EDGE_CURVE('',#8346,#8345,#4960,.T.);
#10726=EDGE_CURVE('',#8347,#8347,#1452,.T.);
#10727=EDGE_CURVE('',#8348,#8348,#1453,.T.);
#10728=EDGE_CURVE('',#8349,#8349,#1454,.T.);
#10729=EDGE_CURVE('',#8349,#8347,#4961,.T.);
#10730=EDGE_CURVE('',#8350,#8350,#1455,.T.);
#10731=EDGE_CURVE('',#8350,#8348,#4962,.T.);
#10732=EDGE_CURVE('',#8346,#8351,#4963,.T.);
#10733=EDGE_CURVE('',#8351,#8352,#4964,.T.);
#10734=EDGE_CURVE('',#8353,#8352,#4965,.T.);
#10735=EDGE_CURVE('',#8354,#8353,#4966,.T.);
#10736=EDGE_CURVE('',#8354,#8344,#4967,.T.);
#10737=EDGE_CURVE('',#8355,#8354,#4968,.T.);
#10738=EDGE_CURVE('',#8355,#8343,#4969,.T.);
#10739=EDGE_CURVE('',#8356,#8357,#4970,.T.);
#10740=EDGE_CURVE('',#8357,#8345,#4971,.T.);
#10741=EDGE_CURVE('',#8358,#8355,#4972,.T.);
#10742=EDGE_CURVE('',#8358,#8356,#4973,.T.);
#10743=EDGE_CURVE('',#8352,#8356,#4974,.T.);
#10744=EDGE_CURVE('',#8353,#8358,#4975,.T.);
#10745=EDGE_CURVE('',#8310,#8359,#4976,.T.);
#10746=EDGE_CURVE('',#8360,#8309,#4977,.T.);
#10747=EDGE_CURVE('',#8359,#8360,#4978,.T.);
#10748=EDGE_CURVE('',#8361,#8362,#4979,.T.);
#10749=EDGE_CURVE('',#8362,#8363,#4980,.T.);
#10750=EDGE_CURVE('',#8363,#8364,#4981,.T.);
#10751=EDGE_CURVE('',#8364,#8365,#4982,.T.);
#10752=EDGE_CURVE('',#8365,#8366,#4983,.T.);
#10753=EDGE_CURVE('',#8366,#8361,#4984,.T.);
#10754=EDGE_CURVE('',#8321,#8313,#4985,.T.);
#10755=EDGE_CURVE('',#8361,#8312,#4986,.T.);
#10756=EDGE_CURVE('',#8366,#8328,#4987,.T.);
#10757=EDGE_CURVE('',#8357,#8314,#4988,.T.);
#10758=EDGE_CURVE('',#8365,#8351,#4989,.T.);
#10759=EDGE_CURVE('',#8351,#8357,#4990,.T.);
#10760=EDGE_CURVE('',#8364,#8300,#4991,.T.);
#10761=EDGE_CURVE('',#8306,#8291,#4992,.T.);
#10762=EDGE_CURVE('',#8296,#8360,#4993,.T.);
#10763=EDGE_CURVE('',#8297,#8359,#4994,.T.);
#10764=EDGE_CURVE('',#8293,#8311,#4995,.T.);
#10765=EDGE_CURVE('',#8305,#8292,#4996,.T.);
#10766=EDGE_CURVE('',#8362,#8304,#4997,.T.);
#10767=EDGE_CURVE('',#8363,#8301,#4998,.T.);
#15064=ORIENTED_EDGE('',*,*,#10584,.F.);
#15065=ORIENTED_EDGE('',*,*,#10585,.T.);
#15066=ORIENTED_EDGE('',*,*,#10586,.T.);
#15067=ORIENTED_EDGE('',*,*,#10585,.F.);
#15068=ORIENTED_EDGE('',*,*,#10587,.T.);
#15069=ORIENTED_EDGE('',*,*,#10588,.T.);
#15070=ORIENTED_EDGE('',*,*,#10589,.T.);
#15071=ORIENTED_EDGE('',*,*,#10590,.F.);
#15072=ORIENTED_EDGE('',*,*,#10589,.F.);
#15073=ORIENTED_EDGE('',*,*,#10591,.T.);
#15074=ORIENTED_EDGE('',*,*,#10592,.T.);
#15075=ORIENTED_EDGE('',*,*,#10591,.F.);
#15076=ORIENTED_EDGE('',*,*,#10588,.F.);
#15077=ORIENTED_EDGE('',*,*,#10593,.F.);
#15078=ORIENTED_EDGE('',*,*,#10594,.F.);
#15079=ORIENTED_EDGE('',*,*,#10595,.F.);
#15080=ORIENTED_EDGE('',*,*,#10596,.F.);
#15081=ORIENTED_EDGE('',*,*,#10597,.F.);
#15082=ORIENTED_EDGE('',*,*,#10598,.F.);
#15083=ORIENTED_EDGE('',*,*,#10599,.F.);
#15084=ORIENTED_EDGE('',*,*,#10600,.F.);
#15085=ORIENTED_EDGE('',*,*,#10594,.T.);
#15086=ORIENTED_EDGE('',*,*,#10601,.T.);
#15087=ORIENTED_EDGE('',*,*,#10602,.F.);
#15088=ORIENTED_EDGE('',*,*,#10603,.F.);
#15089=ORIENTED_EDGE('',*,*,#10595,.T.);
#15090=ORIENTED_EDGE('',*,*,#10600,.T.);
#15091=ORIENTED_EDGE('',*,*,#10604,.F.);
#15092=ORIENTED_EDGE('',*,*,#10605,.F.);
#15093=ORIENTED_EDGE('',*,*,#10596,.T.);
#15094=ORIENTED_EDGE('',*,*,#10603,.T.);
#15095=ORIENTED_EDGE('',*,*,#10606,.F.);
#15096=ORIENTED_EDGE('',*,*,#10607,.F.);
#15097=ORIENTED_EDGE('',*,*,#10597,.T.);
#15098=ORIENTED_EDGE('',*,*,#10605,.T.);
#15099=ORIENTED_EDGE('',*,*,#10608,.F.);
#15100=ORIENTED_EDGE('',*,*,#10609,.F.);
#15101=ORIENTED_EDGE('',*,*,#10598,.T.);
#15102=ORIENTED_EDGE('',*,*,#10607,.T.);
#15103=ORIENTED_EDGE('',*,*,#10610,.F.);
#15104=ORIENTED_EDGE('',*,*,#10601,.F.);
#15105=ORIENTED_EDGE('',*,*,#10593,.T.);
#15106=ORIENTED_EDGE('',*,*,#10609,.T.);
#15107=ORIENTED_EDGE('',*,*,#10611,.F.);
#15108=ORIENTED_EDGE('',*,*,#10612,.F.);
#15109=ORIENTED_EDGE('',*,*,#10613,.F.);
#15110=ORIENTED_EDGE('',*,*,#10614,.F.);
#15111=ORIENTED_EDGE('',*,*,#10615,.F.);
#15112=ORIENTED_EDGE('',*,*,#10616,.F.);
#15113=ORIENTED_EDGE('',*,*,#10617,.F.);
#15114=ORIENTED_EDGE('',*,*,#10618,.F.);
#15115=ORIENTED_EDGE('',*,*,#10619,.F.);
#15116=ORIENTED_EDGE('',*,*,#10620,.F.);
#15117=ORIENTED_EDGE('',*,*,#10621,.F.);
#15118=ORIENTED_EDGE('',*,*,#10622,.F.);
#15119=ORIENTED_EDGE('',*,*,#10623,.F.);
#15120=ORIENTED_EDGE('',*,*,#10624,.F.);
#15121=ORIENTED_EDGE('',*,*,#10612,.T.);
#15122=ORIENTED_EDGE('',*,*,#10625,.T.);
#15123=ORIENTED_EDGE('',*,*,#10626,.F.);
#15124=ORIENTED_EDGE('',*,*,#10627,.F.);
#15125=ORIENTED_EDGE('',*,*,#10613,.T.);
#15126=ORIENTED_EDGE('',*,*,#10624,.T.);
#15127=ORIENTED_EDGE('',*,*,#10628,.F.);
#15128=ORIENTED_EDGE('',*,*,#10629,.F.);
#15129=ORIENTED_EDGE('',*,*,#10614,.T.);
#15130=ORIENTED_EDGE('',*,*,#10627,.T.);
#15131=ORIENTED_EDGE('',*,*,#10630,.F.);
#15132=ORIENTED_EDGE('',*,*,#10631,.F.);
#15133=ORIENTED_EDGE('',*,*,#10615,.T.);
#15134=ORIENTED_EDGE('',*,*,#10629,.T.);
#15135=ORIENTED_EDGE('',*,*,#10632,.F.);
#15136=ORIENTED_EDGE('',*,*,#10633,.F.);
#15137=ORIENTED_EDGE('',*,*,#10616,.T.);
#15138=ORIENTED_EDGE('',*,*,#10631,.T.);
#15139=ORIENTED_EDGE('',*,*,#10634,.F.);
#15140=ORIENTED_EDGE('',*,*,#10635,.F.);
#15141=ORIENTED_EDGE('',*,*,#10617,.T.);
#15142=ORIENTED_EDGE('',*,*,#10633,.T.);
#15143=ORIENTED_EDGE('',*,*,#10636,.F.);
#15144=ORIENTED_EDGE('',*,*,#10637,.F.);
#15145=ORIENTED_EDGE('',*,*,#10618,.T.);
#15146=ORIENTED_EDGE('',*,*,#10635,.T.);
#15147=ORIENTED_EDGE('',*,*,#10638,.F.);
#15148=ORIENTED_EDGE('',*,*,#10639,.F.);
#15149=ORIENTED_EDGE('',*,*,#10619,.T.);
#15150=ORIENTED_EDGE('',*,*,#10637,.T.);
#15151=ORIENTED_EDGE('',*,*,#10640,.F.);
#15152=ORIENTED_EDGE('',*,*,#10641,.F.);
#15153=ORIENTED_EDGE('',*,*,#10620,.T.);
#15154=ORIENTED_EDGE('',*,*,#10639,.T.);
#15155=ORIENTED_EDGE('',*,*,#10642,.F.);
#15156=ORIENTED_EDGE('',*,*,#10643,.F.);
#15157=ORIENTED_EDGE('',*,*,#10621,.T.);
#15158=ORIENTED_EDGE('',*,*,#10641,.T.);
#15159=ORIENTED_EDGE('',*,*,#10644,.F.);
#15160=ORIENTED_EDGE('',*,*,#10645,.F.);
#15161=ORIENTED_EDGE('',*,*,#10622,.T.);
#15162=ORIENTED_EDGE('',*,*,#10643,.T.);
#15163=ORIENTED_EDGE('',*,*,#10646,.F.);
#15164=ORIENTED_EDGE('',*,*,#10625,.F.);
#15165=ORIENTED_EDGE('',*,*,#10611,.T.);
#15166=ORIENTED_EDGE('',*,*,#10645,.T.);
#15167=ORIENTED_EDGE('',*,*,#10647,.F.);
#15168=ORIENTED_EDGE('',*,*,#10648,.F.);
#15169=ORIENTED_EDGE('',*,*,#10649,.T.);
#15170=ORIENTED_EDGE('',*,*,#10650,.T.);
#15171=ORIENTED_EDGE('',*,*,#10651,.F.);
#15172=ORIENTED_EDGE('',*,*,#10652,.F.);
#15173=ORIENTED_EDGE('',*,*,#10653,.F.);
#15174=ORIENTED_EDGE('',*,*,#10647,.T.);
#15175=ORIENTED_EDGE('',*,*,#10654,.F.);
#15176=ORIENTED_EDGE('',*,*,#10655,.F.);
#15177=ORIENTED_EDGE('',*,*,#10656,.F.);
#15178=ORIENTED_EDGE('',*,*,#10652,.T.);
#15179=ORIENTED_EDGE('',*,*,#10657,.F.);
#15180=ORIENTED_EDGE('',*,*,#10658,.F.);
#15181=ORIENTED_EDGE('',*,*,#10659,.F.);
#15182=ORIENTED_EDGE('',*,*,#10660,.T.);
#15183=ORIENTED_EDGE('',*,*,#10661,.F.);
#15184=ORIENTED_EDGE('',*,*,#10662,.F.);
#15185=ORIENTED_EDGE('',*,*,#10663,.F.);
#15186=ORIENTED_EDGE('',*,*,#10658,.T.);
#15187=ORIENTED_EDGE('',*,*,#10664,.F.);
#15188=ORIENTED_EDGE('',*,*,#10665,.T.);
#15189=ORIENTED_EDGE('',*,*,#10666,.F.);
#15190=ORIENTED_EDGE('',*,*,#10667,.F.);
#15191=ORIENTED_EDGE('',*,*,#10662,.T.);
#15192=ORIENTED_EDGE('',*,*,#10668,.F.);
#15193=ORIENTED_EDGE('',*,*,#10669,.F.);
#15194=ORIENTED_EDGE('',*,*,#10670,.F.);
#15195=ORIENTED_EDGE('',*,*,#10671,.F.);
#15196=ORIENTED_EDGE('',*,*,#10672,.F.);
#15197=ORIENTED_EDGE('',*,*,#10673,.T.);
#15198=ORIENTED_EDGE('',*,*,#10674,.F.);
#15199=ORIENTED_EDGE('',*,*,#10675,.F.);
#15200=ORIENTED_EDGE('',*,*,#10676,.F.);
#15201=ORIENTED_EDGE('',*,*,#10669,.T.);
#15202=ORIENTED_EDGE('',*,*,#10677,.F.);
#15203=ORIENTED_EDGE('',*,*,#10678,.T.);
#15204=ORIENTED_EDGE('',*,*,#10679,.T.);
#15205=ORIENTED_EDGE('',*,*,#10680,.T.);
#15206=ORIENTED_EDGE('',*,*,#10681,.T.);
#15207=ORIENTED_EDGE('',*,*,#10678,.F.);
#15208=ORIENTED_EDGE('',*,*,#10681,.F.);
#15209=ORIENTED_EDGE('',*,*,#10682,.T.);
#15210=ORIENTED_EDGE('',*,*,#10683,.T.);
#15211=ORIENTED_EDGE('',*,*,#10679,.F.);
#15212=ORIENTED_EDGE('',*,*,#10683,.F.);
#15213=ORIENTED_EDGE('',*,*,#10684,.T.);
#15214=ORIENTED_EDGE('',*,*,#10685,.T.);
#15215=ORIENTED_EDGE('',*,*,#10686,.T.);
#15216=ORIENTED_EDGE('',*,*,#10687,.F.);
#15217=ORIENTED_EDGE('',*,*,#10688,.F.);
#15218=ORIENTED_EDGE('',*,*,#10689,.T.);
#15219=ORIENTED_EDGE('',*,*,#10690,.T.);
#15220=ORIENTED_EDGE('',*,*,#10689,.F.);
#15221=ORIENTED_EDGE('',*,*,#10691,.F.);
#15222=ORIENTED_EDGE('',*,*,#10692,.T.);
#15223=ORIENTED_EDGE('',*,*,#10693,.T.);
#15224=ORIENTED_EDGE('',*,*,#10694,.T.);
#15225=ORIENTED_EDGE('',*,*,#10695,.T.);
#15226=ORIENTED_EDGE('',*,*,#10692,.F.);
#15227=ORIENTED_EDGE('',*,*,#10696,.F.);
#15228=ORIENTED_EDGE('',*,*,#10697,.T.);
#15229=ORIENTED_EDGE('',*,*,#10698,.T.);
#15230=ORIENTED_EDGE('',*,*,#10697,.F.);
#15231=ORIENTED_EDGE('',*,*,#10699,.F.);
#15232=ORIENTED_EDGE('',*,*,#10687,.T.);
#15233=ORIENTED_EDGE('',*,*,#10699,.T.);
#15234=ORIENTED_EDGE('',*,*,#10696,.T.);
#15235=ORIENTED_EDGE('',*,*,#10691,.T.);
#15236=ORIENTED_EDGE('',*,*,#10688,.T.);
#15237=ORIENTED_EDGE('',*,*,#10680,.F.);
#15238=ORIENTED_EDGE('',*,*,#10682,.F.);
#15239=ORIENTED_EDGE('',*,*,#10700,.F.);
#15240=ORIENTED_EDGE('',*,*,#10685,.F.);
#15241=ORIENTED_EDGE('',*,*,#10701,.F.);
#15242=ORIENTED_EDGE('',*,*,#10694,.F.);
#15243=ORIENTED_EDGE('',*,*,#10702,.F.);
#15244=ORIENTED_EDGE('',*,*,#10703,.F.);
#15245=ORIENTED_EDGE('',*,*,#10704,.F.);
#15246=ORIENTED_EDGE('',*,*,#10705,.F.);
#15247=ORIENTED_EDGE('',*,*,#10706,.T.);
#15248=ORIENTED_EDGE('',*,*,#10707,.T.);
#15249=ORIENTED_EDGE('',*,*,#10708,.T.);
#15250=ORIENTED_EDGE('',*,*,#10709,.T.);
#15251=ORIENTED_EDGE('',*,*,#10710,.T.);
#15252=ORIENTED_EDGE('',*,*,#10711,.T.);
#15253=ORIENTED_EDGE('',*,*,#10712,.F.);
#15254=ORIENTED_EDGE('',*,*,#10713,.F.);
#15255=ORIENTED_EDGE('',*,*,#10695,.F.);
#15256=ORIENTED_EDGE('',*,*,#10714,.F.);
#15257=ORIENTED_EDGE('',*,*,#10711,.F.);
#15258=ORIENTED_EDGE('',*,*,#10715,.T.);
#15259=ORIENTED_EDGE('',*,*,#10703,.T.);
#15260=ORIENTED_EDGE('',*,*,#10716,.F.);
#15261=ORIENTED_EDGE('',*,*,#10684,.F.);
#15262=ORIENTED_EDGE('',*,*,#10690,.F.);
#15263=ORIENTED_EDGE('',*,*,#10713,.T.);
#15264=ORIENTED_EDGE('',*,*,#10717,.T.);
#15265=ORIENTED_EDGE('',*,*,#10707,.F.);
#15266=ORIENTED_EDGE('',*,*,#10717,.F.);
#15267=ORIENTED_EDGE('',*,*,#10712,.T.);
#15268=ORIENTED_EDGE('',*,*,#10718,.T.);
#15269=ORIENTED_EDGE('',*,*,#10706,.F.);
#15270=ORIENTED_EDGE('',*,*,#10718,.F.);
#15271=ORIENTED_EDGE('',*,*,#10704,.T.);
#15272=ORIENTED_EDGE('',*,*,#10715,.F.);
#15273=ORIENTED_EDGE('',*,*,#10710,.F.);
#15274=ORIENTED_EDGE('',*,*,#10719,.T.);
#15275=ORIENTED_EDGE('',*,*,#10587,.F.);
#15276=ORIENTED_EDGE('',*,*,#10590,.T.);
#15277=ORIENTED_EDGE('',*,*,#10720,.F.);
#15278=ORIENTED_EDGE('',*,*,#10721,.T.);
#15279=ORIENTED_EDGE('',*,*,#10722,.T.);
#15280=ORIENTED_EDGE('',*,*,#10705,.T.);
#15281=ORIENTED_EDGE('',*,*,#10719,.F.);
#15282=ORIENTED_EDGE('',*,*,#10709,.F.);
#15283=ORIENTED_EDGE('',*,*,#10723,.T.);
#15284=ORIENTED_EDGE('',*,*,#10724,.F.);
#15285=ORIENTED_EDGE('',*,*,#10702,.T.);
#15286=ORIENTED_EDGE('',*,*,#10722,.F.);
#15287=ORIENTED_EDGE('',*,*,#10725,.F.);
#15288=ORIENTED_EDGE('',*,*,#10723,.F.);
#15289=ORIENTED_EDGE('',*,*,#10708,.F.);
#15290=ORIENTED_EDGE('',*,*,#10714,.T.);
#15291=ORIENTED_EDGE('',*,*,#10701,.T.);
#15292=ORIENTED_EDGE('',*,*,#10716,.T.);
#15293=ORIENTED_EDGE('',*,*,#10726,.T.);
#15294=ORIENTED_EDGE('',*,*,#10592,.F.);
#15295=ORIENTED_EDGE('',*,*,#10727,.T.);
#15296=ORIENTED_EDGE('',*,*,#10586,.F.);
#15297=ORIENTED_EDGE('',*,*,#10728,.T.);
#15298=ORIENTED_EDGE('',*,*,#10729,.T.);
#15299=ORIENTED_EDGE('',*,*,#10726,.F.);
#15300=ORIENTED_EDGE('',*,*,#10729,.F.);
#15301=ORIENTED_EDGE('',*,*,#10730,.T.);
#15302=ORIENTED_EDGE('',*,*,#10731,.T.);
#15303=ORIENTED_EDGE('',*,*,#10727,.F.);
#15304=ORIENTED_EDGE('',*,*,#10731,.F.);
#15305=ORIENTED_EDGE('',*,*,#10724,.T.);
#15306=ORIENTED_EDGE('',*,*,#10732,.T.);
#15307=ORIENTED_EDGE('',*,*,#10733,.T.);
#15308=ORIENTED_EDGE('',*,*,#10734,.F.);
#15309=ORIENTED_EDGE('',*,*,#10735,.F.);
#15310=ORIENTED_EDGE('',*,*,#10736,.T.);
#15311=ORIENTED_EDGE('',*,*,#10720,.T.);
#15312=ORIENTED_EDGE('',*,*,#10736,.F.);
#15313=ORIENTED_EDGE('',*,*,#10737,.F.);
#15314=ORIENTED_EDGE('',*,*,#10738,.T.);
#15315=ORIENTED_EDGE('',*,*,#10739,.T.);
#15316=ORIENTED_EDGE('',*,*,#10740,.T.);
#15317=ORIENTED_EDGE('',*,*,#10721,.F.);
#15318=ORIENTED_EDGE('',*,*,#10738,.F.);
#15319=ORIENTED_EDGE('',*,*,#10741,.F.);
#15320=ORIENTED_EDGE('',*,*,#10742,.T.);
#15321=ORIENTED_EDGE('',*,*,#10743,.T.);
#15322=ORIENTED_EDGE('',*,*,#10742,.F.);
#15323=ORIENTED_EDGE('',*,*,#10744,.F.);
#15324=ORIENTED_EDGE('',*,*,#10734,.T.);
#15325=ORIENTED_EDGE('',*,*,#10744,.T.);
#15326=ORIENTED_EDGE('',*,*,#10741,.T.);
#15327=ORIENTED_EDGE('',*,*,#10737,.T.);
#15328=ORIENTED_EDGE('',*,*,#10735,.T.);
#15329=ORIENTED_EDGE('',*,*,#10728,.F.);
#15330=ORIENTED_EDGE('',*,*,#10730,.F.);
#15331=ORIENTED_EDGE('',*,*,#10745,.F.);
#15332=ORIENTED_EDGE('',*,*,#10671,.T.);
#15333=ORIENTED_EDGE('',*,*,#10746,.F.);
#15334=ORIENTED_EDGE('',*,*,#10747,.F.);
#15335=ORIENTED_EDGE('',*,*,#10748,.T.);
#15336=ORIENTED_EDGE('',*,*,#10749,.T.);
#15337=ORIENTED_EDGE('',*,*,#10750,.T.);
#15338=ORIENTED_EDGE('',*,*,#10751,.T.);
#15339=ORIENTED_EDGE('',*,*,#10752,.T.);
#15340=ORIENTED_EDGE('',*,*,#10753,.T.);
#15341=ORIENTED_EDGE('',*,*,#10754,.T.);
#15342=ORIENTED_EDGE('',*,*,#10674,.T.);
#15343=ORIENTED_EDGE('',*,*,#10755,.F.);
#15344=ORIENTED_EDGE('',*,*,#10753,.F.);
#15345=ORIENTED_EDGE('',*,*,#10756,.T.);
#15346=ORIENTED_EDGE('',*,*,#10693,.F.);
#15347=ORIENTED_EDGE('',*,*,#10698,.F.);
#15348=ORIENTED_EDGE('',*,*,#10686,.F.);
#15349=ORIENTED_EDGE('',*,*,#10757,.T.);
#15350=ORIENTED_EDGE('',*,*,#10675,.T.);
#15351=ORIENTED_EDGE('',*,*,#10754,.F.);
#15352=ORIENTED_EDGE('',*,*,#10700,.T.);
#15353=ORIENTED_EDGE('',*,*,#10756,.F.);
#15354=ORIENTED_EDGE('',*,*,#10752,.F.);
#15355=ORIENTED_EDGE('',*,*,#10758,.T.);
#15356=ORIENTED_EDGE('',*,*,#10759,.T.);
#15357=ORIENTED_EDGE('',*,*,#10584,.T.);
#15358=ORIENTED_EDGE('',*,*,#10760,.T.);
#15359=ORIENTED_EDGE('',*,*,#10659,.T.);
#15360=ORIENTED_EDGE('',*,*,#10663,.T.);
#15361=ORIENTED_EDGE('',*,*,#10667,.T.);
#15362=ORIENTED_EDGE('',*,*,#10761,.T.);
#15363=ORIENTED_EDGE('',*,*,#10648,.T.);
#15364=ORIENTED_EDGE('',*,*,#10653,.T.);
#15365=ORIENTED_EDGE('',*,*,#10656,.T.);
#15366=ORIENTED_EDGE('',*,*,#10762,.T.);
#15367=ORIENTED_EDGE('',*,*,#10746,.T.);
#15368=ORIENTED_EDGE('',*,*,#10670,.T.);
#15369=ORIENTED_EDGE('',*,*,#10676,.T.);
#15370=ORIENTED_EDGE('',*,*,#10757,.F.);
#15371=ORIENTED_EDGE('',*,*,#10739,.F.);
#15372=ORIENTED_EDGE('',*,*,#10743,.F.);
#15373=ORIENTED_EDGE('',*,*,#10733,.F.);
#15374=ORIENTED_EDGE('',*,*,#10758,.F.);
#15375=ORIENTED_EDGE('',*,*,#10751,.F.);
#15376=ORIENTED_EDGE('',*,*,#10762,.F.);
#15377=ORIENTED_EDGE('',*,*,#10655,.T.);
#15378=ORIENTED_EDGE('',*,*,#10763,.T.);
#15379=ORIENTED_EDGE('',*,*,#10747,.T.);
#15380=ORIENTED_EDGE('',*,*,#10763,.F.);
#15381=ORIENTED_EDGE('',*,*,#10657,.T.);
#15382=ORIENTED_EDGE('',*,*,#10654,.T.);
#15383=ORIENTED_EDGE('',*,*,#10651,.T.);
#15384=ORIENTED_EDGE('',*,*,#10764,.T.);
#15385=ORIENTED_EDGE('',*,*,#10677,.T.);
#15386=ORIENTED_EDGE('',*,*,#10672,.T.);
#15387=ORIENTED_EDGE('',*,*,#10745,.T.);
#15388=ORIENTED_EDGE('',*,*,#10765,.F.);
#15389=ORIENTED_EDGE('',*,*,#10665,.F.);
#15390=ORIENTED_EDGE('',*,*,#10766,.F.);
#15391=ORIENTED_EDGE('',*,*,#10748,.F.);
#15392=ORIENTED_EDGE('',*,*,#10755,.T.);
#15393=ORIENTED_EDGE('',*,*,#10673,.F.);
#15394=ORIENTED_EDGE('',*,*,#10764,.F.);
#15395=ORIENTED_EDGE('',*,*,#10650,.F.);
#15396=ORIENTED_EDGE('',*,*,#10732,.F.);
#15397=ORIENTED_EDGE('',*,*,#10725,.T.);
#15398=ORIENTED_EDGE('',*,*,#10740,.F.);
#15399=ORIENTED_EDGE('',*,*,#10759,.F.);
#15400=ORIENTED_EDGE('',*,*,#10767,.T.);
#15401=ORIENTED_EDGE('',*,*,#10660,.F.);
#15402=ORIENTED_EDGE('',*,*,#10760,.F.);
#15403=ORIENTED_EDGE('',*,*,#10750,.F.);
#15404=ORIENTED_EDGE('',*,*,#10766,.T.);
#15405=ORIENTED_EDGE('',*,*,#10668,.T.);
#15406=ORIENTED_EDGE('',*,*,#10664,.T.);
#15407=ORIENTED_EDGE('',*,*,#10661,.T.);
#15408=ORIENTED_EDGE('',*,*,#10767,.F.);
#15409=ORIENTED_EDGE('',*,*,#10749,.F.);
#15410=ORIENTED_EDGE('',*,*,#10666,.T.);
#15411=ORIENTED_EDGE('',*,*,#10765,.T.);
#15412=ORIENTED_EDGE('',*,*,#10649,.F.);
#15413=ORIENTED_EDGE('',*,*,#10761,.F.);
#15414=ORIENTED_EDGE('',*,*,#10610,.T.);
#15415=ORIENTED_EDGE('',*,*,#10608,.T.);
#15416=ORIENTED_EDGE('',*,*,#10606,.T.);
#15417=ORIENTED_EDGE('',*,*,#10604,.T.);
#15418=ORIENTED_EDGE('',*,*,#10602,.T.);
#15419=ORIENTED_EDGE('',*,*,#10599,.T.);
#15420=ORIENTED_EDGE('',*,*,#10646,.T.);
#15421=ORIENTED_EDGE('',*,*,#10644,.T.);
#15422=ORIENTED_EDGE('',*,*,#10642,.T.);
#15423=ORIENTED_EDGE('',*,*,#10640,.T.);
#15424=ORIENTED_EDGE('',*,*,#10638,.T.);
#15425=ORIENTED_EDGE('',*,*,#10636,.T.);
#15426=ORIENTED_EDGE('',*,*,#10634,.T.);
#15427=ORIENTED_EDGE('',*,*,#10632,.T.);
#15428=ORIENTED_EDGE('',*,*,#10630,.T.);
#15429=ORIENTED_EDGE('',*,*,#10628,.T.);
#15430=ORIENTED_EDGE('',*,*,#10626,.T.);
#15431=ORIENTED_EDGE('',*,*,#10623,.T.);
#16713=PLANE('',#19089);
#16714=PLANE('',#19095);
#16715=PLANE('',#19096);
#16716=PLANE('',#19097);
#16717=PLANE('',#19098);
#16718=PLANE('',#19099);
#16719=PLANE('',#19100);
#16720=PLANE('',#19101);
#16721=PLANE('',#19102);
#16722=PLANE('',#19103);
#16723=PLANE('',#19104);
#16724=PLANE('',#19105);
#16725=PLANE('',#19106);
#16726=PLANE('',#19107);
#16727=PLANE('',#19108);
#16728=PLANE('',#19109);
#16729=PLANE('',#19110);
#16730=PLANE('',#19111);
#16731=PLANE('',#19112);
#16732=PLANE('',#19113);
#16733=PLANE('',#19114);
#16734=PLANE('',#19115);
#16735=PLANE('',#19116);
#16736=PLANE('',#19117);
#16737=PLANE('',#19119);
#16738=PLANE('',#19125);
#16739=PLANE('',#19126);
#16740=PLANE('',#19127);
#16741=PLANE('',#19128);
#16742=PLANE('',#19129);
#16743=PLANE('',#19130);
#16744=PLANE('',#19131);
#16745=PLANE('',#19134);
#16746=PLANE('',#19137);
#16747=PLANE('',#19140);
#16748=PLANE('',#19141);
#16749=PLANE('',#19142);
#16750=PLANE('',#19143);
#16751=PLANE('',#19145);
#16752=PLANE('',#19151);
#16753=PLANE('',#19152);
#16754=PLANE('',#19153);
#16755=PLANE('',#19154);
#16756=PLANE('',#19155);
#16757=PLANE('',#19156);
#16758=PLANE('',#19157);
#16759=PLANE('',#19158);
#16760=PLANE('',#19159);
#16761=PLANE('',#19160);
#16762=PLANE('',#19161);
#16763=PLANE('',#19162);
#16764=PLANE('',#19163);
#16765=PLANE('',#19164);
#16766=PLANE('',#19165);
#16767=PLANE('',#19166);
#16768=PLANE('',#19167);
#17552=ADVANCED_FACE('',(#2217),#702,.F.);
#17553=ADVANCED_FACE('',(#2218),#16713,.T.);
#17554=ADVANCED_FACE('',(#2219),#703,.F.);
#17555=ADVANCED_FACE('',(#2220),#16714,.F.);
#17556=ADVANCED_FACE('',(#2221),#16715,.T.);
#17557=ADVANCED_FACE('',(#2222),#16716,.T.);
#17558=ADVANCED_FACE('',(#2223),#16717,.T.);
#17559=ADVANCED_FACE('',(#2224),#16718,.T.);
#17560=ADVANCED_FACE('',(#2225),#16719,.T.);
#17561=ADVANCED_FACE('',(#2226),#16720,.T.);
#17562=ADVANCED_FACE('',(#2227),#16721,.F.);
#17563=ADVANCED_FACE('',(#2228),#53,.T.);
#17564=ADVANCED_FACE('',(#2229),#54,.T.);
#17565=ADVANCED_FACE('',(#2230),#16722,.T.);
#17566=ADVANCED_FACE('',(#2231),#16723,.T.);
#17567=ADVANCED_FACE('',(#2232),#16724,.T.);
#17568=ADVANCED_FACE('',(#2233),#16725,.T.);
#17569=ADVANCED_FACE('',(#2234),#16726,.T.);
#17570=ADVANCED_FACE('',(#2235),#55,.T.);
#17571=ADVANCED_FACE('',(#2236),#56,.T.);
#17572=ADVANCED_FACE('',(#2237),#57,.T.);
#17573=ADVANCED_FACE('',(#2238),#16727,.T.);
#17574=ADVANCED_FACE('',(#2239),#58,.T.);
#17575=ADVANCED_FACE('',(#2240),#16728,.F.);
#17576=ADVANCED_FACE('',(#2241),#16729,.F.);
#17577=ADVANCED_FACE('',(#2242),#16730,.F.);
#17578=ADVANCED_FACE('',(#2243),#16731,.F.);
#17579=ADVANCED_FACE('',(#2244),#16732,.F.);
#17580=ADVANCED_FACE('',(#2245),#16733,.F.);
#17581=ADVANCED_FACE('',(#2246),#16734,.F.);
#17582=ADVANCED_FACE('',(#2247),#16735,.F.);
#17583=ADVANCED_FACE('',(#2248),#16736,.F.);
#17584=ADVANCED_FACE('',(#2249),#16737,.F.);
#17585=ADVANCED_FACE('',(#2250),#704,.F.);
#17586=ADVANCED_FACE('',(#2251),#705,.F.);
#17587=ADVANCED_FACE('',(#2252),#16738,.F.);
#17588=ADVANCED_FACE('',(#2253),#16739,.F.);
#17589=ADVANCED_FACE('',(#2254),#16740,.F.);
#17590=ADVANCED_FACE('',(#2255),#16741,.F.);
#17591=ADVANCED_FACE('',(#2256,#942,#943),#16742,.F.);
#17592=ADVANCED_FACE('',(#2257),#16743,.T.);
#17593=ADVANCED_FACE('',(#2258,#944,#945),#16744,.F.);
#17594=ADVANCED_FACE('',(#2259,#946,#947),#16745,.T.);
#17595=ADVANCED_FACE('',(#2260),#16746,.F.);
#17596=ADVANCED_FACE('',(#2261),#706,.F.);
#17597=ADVANCED_FACE('',(#2262),#707,.F.);
#17598=ADVANCED_FACE('',(#2263,#948),#16747,.F.);
#17599=ADVANCED_FACE('',(#2264),#16748,.F.);
#17600=ADVANCED_FACE('',(#2265),#16749,.F.);
#17601=ADVANCED_FACE('',(#2266,#949),#16750,.F.);
#17602=ADVANCED_FACE('',(#2267,#950),#16751,.F.);
#17603=ADVANCED_FACE('',(#2268),#708,.F.);
#17604=ADVANCED_FACE('',(#2269),#709,.F.);
#17605=ADVANCED_FACE('',(#2270),#16752,.F.);
#17606=ADVANCED_FACE('',(#2271),#16753,.F.);
#17607=ADVANCED_FACE('',(#2272),#16754,.F.);
#17608=ADVANCED_FACE('',(#2273),#16755,.F.);
#17609=ADVANCED_FACE('',(#2274,#951,#952),#16756,.F.);
#17610=ADVANCED_FACE('',(#2275),#16757,.F.);
#17611=ADVANCED_FACE('',(#2276),#16758,.T.);
#17612=ADVANCED_FACE('',(#2277),#16759,.F.);
#17613=ADVANCED_FACE('',(#2278,#953),#16760,.F.);
#17614=ADVANCED_FACE('',(#2279),#16761,.F.);
#17615=ADVANCED_FACE('',(#2280),#16762,.F.);
#17616=ADVANCED_FACE('',(#2281),#16763,.F.);
#17617=ADVANCED_FACE('',(#2282),#16764,.F.);
#17618=ADVANCED_FACE('',(#2283),#16765,.T.);
#17619=ADVANCED_FACE('',(#2284),#16766,.F.);
#17620=ADVANCED_FACE('',(#2285),#16767,.F.);
#17621=ADVANCED_FACE('',(#2286,#954,#955),#16768,.F.);
#17800=CLOSED_SHELL('',(#17552,#17553,#17554,#17555,#17556,#17557,#17558,
#17559,#17560,#17561,#17562,#17563,#17564,#17565,#17566,#17567,#17568,#17569,
#17570,#17571,#17572,#17573,#17574,#17575,#17576,#17577,#17578,#17579,#17580,
#17581,#17582,#17583,#17584,#17585,#17586,#17587,#17588,#17589,#17590,#17591,
#17592,#17593,#17594,#17595,#17596,#17597,#17598,#17599,#17600,#17601,#17602,
#17603,#17604,#17605,#17606,#17607,#17608,#17609,#17610,#17611,#17612,#17613,
#17614,#17615,#17616,#17617,#17618,#17619,#17620,#17621));
#19085=AXIS2_PLACEMENT_3D('',#32971,#23037,#23038);
#19086=AXIS2_PLACEMENT_3D('',#32972,#23039,#23040);
#19087=AXIS2_PLACEMENT_3D('',#32974,#23041,#23042);
#19088=AXIS2_PLACEMENT_3D('',#32977,#23044,#23045);
#19089=AXIS2_PLACEMENT_3D('',#32978,#23046,#23047);
#19090=AXIS2_PLACEMENT_3D('',#32983,#23049,#23050);
#19091=AXIS2_PLACEMENT_3D('',#32984,#23051,#23052);
#19092=AXIS2_PLACEMENT_3D('',#32985,#23053,#23054);
#19093=AXIS2_PLACEMENT_3D('',#32986,#23055,#23056);
#19094=AXIS2_PLACEMENT_3D('',#32989,#23058,#23059);
#19095=AXIS2_PLACEMENT_3D('',#32990,#23060,#23061);
#19096=AXIS2_PLACEMENT_3D('',#33003,#23068,#23069);
#19097=AXIS2_PLACEMENT_3D('',#33009,#23073,#23074);
#19098=AXIS2_PLACEMENT_3D('',#33013,#23077,#23078);
#19099=AXIS2_PLACEMENT_3D('',#33017,#23081,#23082);
#19100=AXIS2_PLACEMENT_3D('',#33021,#23085,#23086);
#19101=AXIS2_PLACEMENT_3D('',#33025,#23089,#23090);
#19102=AXIS2_PLACEMENT_3D('',#33027,#23092,#23093);
#19103=AXIS2_PLACEMENT_3D('',#33260,#23103,#23104);
#19104=AXIS2_PLACEMENT_3D('',#33264,#23107,#23108);
#19105=AXIS2_PLACEMENT_3D('',#33268,#23111,#23112);
#19106=AXIS2_PLACEMENT_3D('',#33272,#23115,#23116);
#19107=AXIS2_PLACEMENT_3D('',#33276,#23119,#23120);
#19108=AXIS2_PLACEMENT_3D('',#33445,#23126,#23127);
#19109=AXIS2_PLACEMENT_3D('',#33506,#23130,#23131);
#19110=AXIS2_PLACEMENT_3D('',#33517,#23137,#23138);
#19111=AXIS2_PLACEMENT_3D('',#33523,#23142,#23143);
#19112=AXIS2_PLACEMENT_3D('',#33529,#23147,#23148);
#19113=AXIS2_PLACEMENT_3D('',#33538,#23153,#23154);
#19114=AXIS2_PLACEMENT_3D('',#33544,#23158,#23159);
#19115=AXIS2_PLACEMENT_3D('',#33552,#23164,#23165);
#19116=AXIS2_PLACEMENT_3D('',#33561,#23170,#23171);
#19117=AXIS2_PLACEMENT_3D('',#33571,#23177,#23178);
#19118=AXIS2_PLACEMENT_3D('',#33573,#23179,#23180);
#19119=AXIS2_PLACEMENT_3D('',#33574,#23181,#23182);
#19120=AXIS2_PLACEMENT_3D('',#33576,#23183,#23184);
#19121=AXIS2_PLACEMENT_3D('',#33577,#23185,#23186);
#19122=AXIS2_PLACEMENT_3D('',#33579,#23187,#23188);
#19123=AXIS2_PLACEMENT_3D('',#33581,#23190,#23191);
#19124=AXIS2_PLACEMENT_3D('',#33583,#23192,#23193);
#19125=AXIS2_PLACEMENT_3D('',#33585,#23195,#23196);
#19126=AXIS2_PLACEMENT_3D('',#33598,#23203,#23204);
#19127=AXIS2_PLACEMENT_3D('',#33604,#23208,#23209);
#19128=AXIS2_PLACEMENT_3D('',#33614,#23215,#23216);
#19129=AXIS2_PLACEMENT_3D('',#33617,#23219,#23220);
#19130=AXIS2_PLACEMENT_3D('',#33618,#23221,#23222);
#19131=AXIS2_PLACEMENT_3D('',#33621,#23225,#23226);
#19132=AXIS2_PLACEMENT_3D('',#33631,#23231,#23232);
#19133=AXIS2_PLACEMENT_3D('',#33633,#23233,#23234);
#19134=AXIS2_PLACEMENT_3D('',#33634,#23235,#23236);
#19135=AXIS2_PLACEMENT_3D('',#33644,#23241,#23242);
#19136=AXIS2_PLACEMENT_3D('',#33646,#23243,#23244);
#19137=AXIS2_PLACEMENT_3D('',#33647,#23245,#23246);
#19138=AXIS2_PLACEMENT_3D('',#33651,#23250,#23251);
#19139=AXIS2_PLACEMENT_3D('',#33653,#23253,#23254);
#19140=AXIS2_PLACEMENT_3D('',#33655,#23256,#23257);
#19141=AXIS2_PLACEMENT_3D('',#33657,#23259,#23260);
#19142=AXIS2_PLACEMENT_3D('',#33667,#23266,#23267);
#19143=AXIS2_PLACEMENT_3D('',#33669,#23269,#23270);
#19144=AXIS2_PLACEMENT_3D('',#33671,#23271,#23272);
#19145=AXIS2_PLACEMENT_3D('',#33672,#23273,#23274);
#19146=AXIS2_PLACEMENT_3D('',#33674,#23275,#23276);
#19147=AXIS2_PLACEMENT_3D('',#33675,#23277,#23278);
#19148=AXIS2_PLACEMENT_3D('',#33677,#23279,#23280);
#19149=AXIS2_PLACEMENT_3D('',#33679,#23282,#23283);
#19150=AXIS2_PLACEMENT_3D('',#33681,#23284,#23285);
#19151=AXIS2_PLACEMENT_3D('',#33683,#23287,#23288);
#19152=AXIS2_PLACEMENT_3D('',#33693,#23294,#23295);
#19153=AXIS2_PLACEMENT_3D('',#33697,#23298,#23299);
#19154=AXIS2_PLACEMENT_3D('',#33705,#23304,#23305);
#19155=AXIS2_PLACEMENT_3D('',#33708,#23308,#23309);
#19156=AXIS2_PLACEMENT_3D('',#33709,#23310,#23311);
#19157=AXIS2_PLACEMENT_3D('',#33715,#23315,#23316);
#19158=AXIS2_PLACEMENT_3D('',#33728,#23323,#23324);
#19159=AXIS2_PLACEMENT_3D('',#33732,#23328,#23329);
#19160=AXIS2_PLACEMENT_3D('',#33736,#23333,#23334);
#19161=AXIS2_PLACEMENT_3D('',#33740,#23338,#23339);
#19162=AXIS2_PLACEMENT_3D('',#33742,#23341,#23342);
#19163=AXIS2_PLACEMENT_3D('',#33744,#23344,#23345);
#19164=AXIS2_PLACEMENT_3D('',#33747,#23348,#23349);
#19165=AXIS2_PLACEMENT_3D('',#33748,#23350,#23351);
#19166=AXIS2_PLACEMENT_3D('',#33750,#23353,#23354);
#19167=AXIS2_PLACEMENT_3D('',#33751,#23355,#23356);
#23037=DIRECTION('axis',(0.,0.,1.));
#23038=DIRECTION('refdir',(1.,0.,0.));
#23039=DIRECTION('center_axis',(0.678851252797501,0.734275817779166,-4.75195876958251E-15));
#23040=DIRECTION('ref_axis',(0.734275817779166,-0.678851252797501,1.00517519845672E-30));
#23041=DIRECTION('center_axis',(0.,1.,4.75809867696506E-15));
#23042=DIRECTION('ref_axis',(1.,-3.06753290551076E-28,6.44697202342886E-14));
#23043=DIRECTION('',(0.678851252797501,0.734275817779166,-4.75195876958251E-15));
#23044=DIRECTION('center_axis',(0.678851252797501,0.734275817779166,-4.75195876958251E-15));
#23045=DIRECTION('ref_axis',(0.734275817779166,-0.678851252797501,1.00517519845672E-30));
#23046=DIRECTION('center_axis',(0.678851252797501,0.734275817779166,-4.75195876958251E-15));
#23047=DIRECTION('ref_axis',(-7.E-15,-1.94922383908984E-32,-1.));
#23048=DIRECTION('',(-7.E-15,0.,-1.));
#23049=DIRECTION('center_axis',(0.678851252797502,0.734275817779166,-4.75195876958251E-15));
#23050=DIRECTION('ref_axis',(0.734275817779166,-0.678851252797502,-4.32833613893531E-30));
#23051=DIRECTION('center_axis',(0.678851252797502,0.734275817779166,-4.75195876958251E-15));
#23052=DIRECTION('ref_axis',(0.734275817779166,-0.678851252797502,-4.32833613893531E-30));
#23053=DIRECTION('center_axis',(0.678851252797502,0.734275817779166,-4.75195876958251E-15));
#23054=DIRECTION('ref_axis',(0.734275817779166,-0.678851252797502,-4.32833613893531E-30));
#23055=DIRECTION('center_axis',(-2.31577568721337E-14,1.,3.10052035742355E-14));
#23056=DIRECTION('ref_axis',(1.,2.31577568721319E-14,6.0898447202096E-14));
#23057=DIRECTION('',(0.678851252797502,0.734275817779166,-4.75195876958251E-15));
#23058=DIRECTION('center_axis',(0.678851252797502,0.734275817779166,-4.75195876958251E-15));
#23059=DIRECTION('ref_axis',(0.734275817779166,-0.678851252797502,-4.32833613893531E-30));
#23060=DIRECTION('center_axis',(-9.66488793758498E-15,-1.,6.76542155630949E-29));
#23061=DIRECTION('ref_axis',(7.E-15,6.6510029763507E-46,1.));
#23062=DIRECTION('',(0.867930013859714,-8.38844632162069E-15,0.496686511837674));
#23063=DIRECTION('',(-7.E-15,0.,-1.));
#23064=DIRECTION('',(1.,-9.94102759294464E-15,-7.E-15));
#23065=DIRECTION('',(-7.E-15,0.,-1.));
#23066=DIRECTION('',(-1.,9.91270557701032E-15,7.E-15));
#23067=DIRECTION('',(7.E-15,0.,1.));
#23068=DIRECTION('center_axis',(1.,-9.98518434391482E-15,-7.E-15));
#23069=DIRECTION('ref_axis',(9.98518434391482E-15,1.,-6.98962904074038E-29));
#23070=DIRECTION('',(-7.E-15,0.,-1.));
#23071=DIRECTION('',(9.98518434391482E-15,1.,-6.98962904074038E-29));
#23072=DIRECTION('',(9.98518434391482E-15,1.,-6.98962904074038E-29));
#23073=DIRECTION('center_axis',(7.E-15,0.,1.));
#23074=DIRECTION('ref_axis',(0.,-1.,0.));
#23075=DIRECTION('',(1.,-9.94102759294464E-15,-7.E-15));
#23076=DIRECTION('',(9.98518434391482E-15,1.,-6.98962904074038E-29));
#23077=DIRECTION('center_axis',(1.,-9.98518434391482E-15,-7.E-15));
#23078=DIRECTION('ref_axis',(9.98518434391482E-15,1.,-6.98962904074038E-29));
#23079=DIRECTION('',(-7.E-15,0.,-1.));
#23080=DIRECTION('',(9.98518434391482E-15,1.,-6.98962904074038E-29));
#23081=DIRECTION('center_axis',(-7.E-15,0.,-1.));
#23082=DIRECTION('ref_axis',(-1.,0.,7.E-15));
#23083=DIRECTION('',(-1.,9.91270557701032E-15,7.E-15));
#23084=DIRECTION('',(9.98518434391482E-15,1.,-6.98962904074038E-29));
#23085=DIRECTION('center_axis',(-1.,9.98518434391482E-15,7.E-15));
#23086=DIRECTION('ref_axis',(9.98518434391482E-15,1.,-6.98962904074038E-29));
#23087=DIRECTION('',(7.E-15,0.,1.));
#23088=DIRECTION('',(9.98518434391482E-15,1.,-6.98962904074038E-29));
#23089=DIRECTION('center_axis',(-0.496686511837674,4.95950638183526E-15,
0.867930013859714));
#23090=DIRECTION('ref_axis',(3.98299326130898E-29,-1.,5.71417775931055E-15));
#23091=DIRECTION('',(0.867930013859714,-8.38844632162069E-15,0.496686511837674));
#23092=DIRECTION('center_axis',(4.21032245990148E-13,-1.,-1.056234085578E-14));
#23093=DIRECTION('ref_axis',(1.,4.21032245990149E-13,-7.E-15));
#23094=DIRECTION('',(0.729691385153428,-6.99094164349059E-15,0.683776631973389));
#23095=DIRECTION('',(-7.E-15,0.,-1.));
#23096=DIRECTION('',(-1.,9.66488793758498E-15,7.E-15));
#23097=DIRECTION('',(7.E-15,0.,1.));
#23098=DIRECTION('',(-0.729724964678349,8.12675361862801E-15,-0.683740795861402));
#23099=DIRECTION('',(-7.E-15,0.,-1.));
#23100=DIRECTION('',(9.98518434391482E-15,1.,-6.98962904074038E-29));
#23101=DIRECTION('',(9.98518434391482E-15,1.,-6.98962904074038E-29));
#23102=DIRECTION('',(9.98518434391482E-15,1.,-6.98962904074038E-29));
#23103=DIRECTION('center_axis',(-0.683776631973389,6.82763572031554E-15,
0.729691385153428));
#23104=DIRECTION('ref_axis',(6.59723735469024E-29,-1.,9.35688136002864E-15));
#23105=DIRECTION('',(0.729691385153428,-6.99094164349059E-15,0.683776631973389));
#23106=DIRECTION('',(9.98518434391482E-15,1.,-6.98962904074038E-29));
#23107=DIRECTION('center_axis',(1.,-9.98518434391482E-15,-7.E-15));
#23108=DIRECTION('ref_axis',(9.98518434391482E-15,1.,-6.98962904074038E-29));
#23109=DIRECTION('',(-7.E-15,0.,-1.));
#23110=DIRECTION('',(9.98518434391482E-15,1.,-6.98962904074038E-29));
#23111=DIRECTION('center_axis',(-7.E-15,0.,-1.));
#23112=DIRECTION('ref_axis',(-1.,0.,7.E-15));
#23113=DIRECTION('',(-1.,9.66488793758498E-15,7.E-15));
#23114=DIRECTION('',(9.98518434391482E-15,1.,-6.98962904074038E-29));
#23115=DIRECTION('center_axis',(-1.,9.98518434391482E-15,7.E-15));
#23116=DIRECTION('ref_axis',(9.98518434391482E-15,1.,-6.98962904074038E-29));
#23117=DIRECTION('',(7.E-15,0.,1.));
#23118=DIRECTION('',(9.98518434391482E-15,1.,-6.98962904074038E-29));
#23119=DIRECTION('center_axis',(0.683740795861402,-6.82727789013118E-15,
-0.729724964678349));
#23120=DIRECTION('ref_axis',(9.98518434391482E-15,1.,-6.960711119349E-29));
#23121=DIRECTION('',(-0.729724964678349,8.12675361862801E-15,-0.683740795861402));
#23122=DIRECTION('',(9.98518434391482E-15,1.,-6.98962904074038E-29));
#23123=DIRECTION('',(9.98518434391482E-15,1.,-6.98962904074038E-29));
#23124=DIRECTION('',(9.98518434391482E-15,1.,-6.98962904074038E-29));
#23125=DIRECTION('',(9.98518434391482E-15,1.,-6.98962904074038E-29));
#23126=DIRECTION('center_axis',(1.,-9.98518434391482E-15,-7.E-15));
#23127=DIRECTION('ref_axis',(9.98518434391482E-15,1.,-6.98962904074038E-29));
#23128=DIRECTION('',(-7.E-15,0.,-1.));
#23129=DIRECTION('',(9.98518434391482E-15,1.,-6.98962904074038E-29));
#23130=DIRECTION('center_axis',(7.E-15,0.,1.));
#23131=DIRECTION('ref_axis',(0.,-1.,0.));
#23132=DIRECTION('',(-1.,9.98518434391482E-15,7.E-15));
#23133=DIRECTION('',(-0.734275817779166,0.678851252797501,5.13993072445416E-15));
#23134=DIRECTION('',(-1.,9.98518434391482E-15,7.E-15));
#23135=DIRECTION('',(1.26416333906609E-14,1.,-8.84914337346266E-29));
#23136=DIRECTION('',(-0.774336703951836,-0.632773789685546,5.42035692766285E-15));
#23137=DIRECTION('center_axis',(-9.98518434391482E-15,-1.,6.98962904074038E-29));
#23138=DIRECTION('ref_axis',(7.E-15,1.46992422332527E-45,1.));
#23139=DIRECTION('',(-1.,9.98518434391482E-15,7.E-15));
#23140=DIRECTION('',(7.E-15,0.,1.));
#23141=DIRECTION('',(-7.E-15,0.,-1.));
#23142=DIRECTION('center_axis',(7.E-15,0.,1.));
#23143=DIRECTION('ref_axis',(0.,-1.,0.));
#23144=DIRECTION('',(-1.,9.98518434391482E-15,7.E-15));
#23145=DIRECTION('',(-0.734275817779166,0.678851252797501,5.13993072445416E-15));
#23146=DIRECTION('',(-0.774336703951836,-0.632773789685546,5.42035692766285E-15));
#23147=DIRECTION('center_axis',(-7.E-15,0.,-1.));
#23148=DIRECTION('ref_axis',(-1.,0.,7.E-15));
#23149=DIRECTION('',(-1.,9.98518434391482E-15,7.E-15));
#23150=DIRECTION('',(0.734275817779166,-0.678851252797501,-5.13993072445416E-15));
#23151=DIRECTION('',(-1.,9.98518434391482E-15,7.E-15));
#23152=DIRECTION('',(0.774336703951836,0.632773789685546,-5.42035692766285E-15));
#23153=DIRECTION('center_axis',(-9.98518434391482E-15,-1.,6.98962904074038E-29));
#23154=DIRECTION('ref_axis',(7.E-15,1.46992422332527E-45,1.));
#23155=DIRECTION('',(-1.,9.98518434391482E-15,7.E-15));
#23156=DIRECTION('',(7.E-15,0.,1.));
#23157=DIRECTION('',(-7.E-15,0.,-1.));
#23158=DIRECTION('center_axis',(-7.E-15,0.,-1.));
#23159=DIRECTION('ref_axis',(-1.,0.,7.E-15));
#23160=DIRECTION('',(-1.25743561522893E-14,-1.,8.8020493066025E-29));
#23161=DIRECTION('',(-1.,9.98518434391482E-15,7.E-15));
#23162=DIRECTION('',(0.734275817779166,-0.678851252797501,-5.13993072445416E-15));
#23163=DIRECTION('',(0.774336703951836,0.632773789685546,-5.42035692766285E-15));
#23164=DIRECTION('center_axis',(9.98518434391482E-15,1.,-6.98962904074038E-29));
#23165=DIRECTION('ref_axis',(-1.,9.98518434391482E-15,7.E-15));
#23166=DIRECTION('',(-1.,9.98518434391482E-15,7.E-15));
#23167=DIRECTION('',(-7.E-15,0.,-1.));
#23168=DIRECTION('',(1.,-9.98518434391482E-15,-7.E-15));
#23169=DIRECTION('',(7.E-15,0.,1.));
#23170=DIRECTION('center_axis',(-7.E-15,3.89480588105756E-17,-1.));
#23171=DIRECTION('ref_axis',(-2.7263641167403E-31,-1.,-3.89480588105756E-17));
#23172=DIRECTION('',(-9.97070305550737E-15,-1.,-3.89480588105058E-17));
#23173=DIRECTION('',(-0.734275817779168,0.6788512527975,5.16637066297176E-15));
#23174=DIRECTION('',(-1.,9.98518434391482E-15,7.E-15));
#23175=DIRECTION('',(0.734275817779166,-0.678851252797501,-5.16637066297175E-15));
#23176=DIRECTION('',(0.774336703951836,0.632773789685546,-5.39571161688839E-15));
#23177=DIRECTION('center_axis',(0.678851252797502,0.734275817779166,-4.75195876958251E-15));
#23178=DIRECTION('ref_axis',(-7.E-15,-2.38284042329043E-31,-1.));
#23179=DIRECTION('center_axis',(-0.678851252797498,-0.734275817779169,4.75195876958249E-15));
#23180=DIRECTION('ref_axis',(-0.734275817779169,0.678851252797498,5.15362541093228E-30));
#23181=DIRECTION('center_axis',(0.6788512527975,0.734275817779167,-4.7519587695825E-15));
#23182=DIRECTION('ref_axis',(-7.E-15,5.87886466093466E-32,-1.));
#23183=DIRECTION('center_axis',(-0.678851252797499,-0.734275817779168,4.75195876958249E-15));
#23184=DIRECTION('ref_axis',(-0.734275817779168,0.678851252797499,2.2007191422899E-30));
#23185=DIRECTION('center_axis',(0.678851252797498,0.734275817779169,-4.75195876958249E-15));
#23186=DIRECTION('ref_axis',(0.734275817779169,-0.678851252797498,8.97702189582066E-30));
#23187=DIRECTION('center_axis',(-0.678851252797501,-0.734275817779167,4.75195876958251E-15));
#23188=DIRECTION('ref_axis',(-0.734275817779167,0.678851252797501,-1.38511036298352E-31));
#23189=DIRECTION('',(0.678851252797498,0.734275817779169,-4.75195876958249E-15));
#23190=DIRECTION('center_axis',(0.678851252797499,0.734275817779168,-4.75195876958249E-15));
#23191=DIRECTION('ref_axis',(0.734275817779168,-0.678851252797499,-2.2007191422899E-30));
#23192=DIRECTION('center_axis',(-0.678851252797499,-0.734275817779168,4.75195876958249E-15));
#23193=DIRECTION('ref_axis',(-0.734275817779168,0.678851252797499,2.2007191422899E-30));
#23194=DIRECTION('',(0.678851252797499,0.734275817779168,-4.75195876958249E-15));
#23195=DIRECTION('center_axis',(-6.91154406257336E-15,-8.17791114530617E-17,
-1.));
#23196=DIRECTION('ref_axis',(-1.,-1.87889345193385E-47,6.91154406257336E-15));
#23197=DIRECTION('',(-0.734275817779168,0.6788512527975,5.01946381640023E-15));
#23198=DIRECTION('',(-0.734275817779168,0.6788512527975,5.01946381640023E-15));
#23199=DIRECTION('',(-0.734275817779168,0.6788512527975,5.01946381640023E-15));
#23200=DIRECTION('',(0.6788512527975,0.734275817779168,-4.7519587695825E-15));
#23201=DIRECTION('',(-0.734275817779168,0.6788512527975,5.01946381640023E-15));
#23202=DIRECTION('',(0.6788512527975,0.734275817779168,-4.7519587695825E-15));
#23203=DIRECTION('center_axis',(-0.734275817779168,0.6788512527975,5.13993072445417E-15));
#23204=DIRECTION('ref_axis',(7.E-15,9.60729613809447E-32,1.));
#23205=DIRECTION('',(7.E-15,0.,1.));
#23206=DIRECTION('',(7.E-15,0.,1.));
#23207=DIRECTION('',(0.6788512527975,0.734275817779168,-4.7519587695825E-15));
#23208=DIRECTION('center_axis',(6.90564700007825E-15,8.72310522165992E-17,
1.));
#23209=DIRECTION('ref_axis',(6.10617365516194E-31,-1.,8.72310522165992E-17));
#23210=DIRECTION('',(0.734275817779168,-0.6788512527975,-5.01143268919663E-15));
#23211=DIRECTION('',(0.734275817779168,-0.6788512527975,-5.01143268919663E-15));
#23212=DIRECTION('',(0.734275817779166,-0.678851252797502,-5.01143268919662E-15));
#23213=DIRECTION('',(0.734275817779168,-0.6788512527975,-5.01143268919663E-15));
#23214=DIRECTION('',(0.6788512527975,0.734275817779168,-4.7519587695825E-15));
#23215=DIRECTION('center_axis',(0.734275817779168,-0.6788512527975,-5.13993072445417E-15));
#23216=DIRECTION('ref_axis',(0.6788512527975,0.734275817779168,-4.7519587695825E-15));
#23217=DIRECTION('',(-7.E-15,0.,-1.));
#23218=DIRECTION('',(-7.E-15,0.,-1.));
#23219=DIRECTION('center_axis',(0.6788512527975,0.734275817779168,-4.7519587695825E-15));
#23220=DIRECTION('ref_axis',(-7.E-15,1.36491689365732E-31,-1.));
#23221=DIRECTION('center_axis',(0.6788512527975,0.734275817779168,-4.7519587695825E-15));
#23222=DIRECTION('ref_axis',(-7.E-15,1.36491689365732E-31,-1.));
#23223=DIRECTION('',(-7.E-15,0.,-1.));
#23224=DIRECTION('',(7.E-15,0.,1.));
#23225=DIRECTION('center_axis',(-7.E-15,0.,-1.));
#23226=DIRECTION('ref_axis',(-1.,0.,7.E-15));
#23227=DIRECTION('',(1.,-2.32761274233658E-16,-7.E-15));
#23228=DIRECTION('',(-0.734275817779166,0.678851252797502,5.13993072445416E-15));
#23229=DIRECTION('',(-1.,0.,7.E-15));
#23230=DIRECTION('',(0.734275817779166,-0.678851252797501,-5.13993072445416E-15));
#23231=DIRECTION('center_axis',(-7.E-15,0.,-1.));
#23232=DIRECTION('ref_axis',(-1.,0.,7.E-15));
#23233=DIRECTION('center_axis',(-7.E-15,0.,-1.));
#23234=DIRECTION('ref_axis',(-1.,0.,7.E-15));
#23235=DIRECTION('center_axis',(-7.E-15,0.,-1.));
#23236=DIRECTION('ref_axis',(-1.,0.,7.E-15));
#23237=DIRECTION('',(1.,-2.32761274233658E-16,-7.E-15));
#23238=DIRECTION('',(0.734275817779166,-0.678851252797501,-5.13993072445416E-15));
#23239=DIRECTION('',(-1.,0.,7.E-15));
#23240=DIRECTION('',(-0.734275817779166,0.678851252797502,5.13993072445416E-15));
#23241=DIRECTION('center_axis',(-7.E-15,0.,-1.));
#23242=DIRECTION('ref_axis',(-1.,0.,7.E-15));
#23243=DIRECTION('center_axis',(-7.E-15,0.,-1.));
#23244=DIRECTION('ref_axis',(-1.,0.,7.E-15));
#23245=DIRECTION('center_axis',(0.678851252797502,0.734275817779166,-4.75195876958251E-15));
#23246=DIRECTION('ref_axis',(-7.E-15,-2.38284042329043E-31,-1.));
#23247=DIRECTION('',(7.E-15,0.,1.));
#23248=DIRECTION('',(7.E-15,0.,1.));
#23249=DIRECTION('',(7.E-15,0.,1.));
#23250=DIRECTION('center_axis',(7.E-15,0.,1.));
#23251=DIRECTION('ref_axis',(1.,0.,-7.E-15));
#23252=DIRECTION('',(7.E-15,0.,1.));
#23253=DIRECTION('center_axis',(7.E-15,0.,1.));
#23254=DIRECTION('ref_axis',(1.,0.,-7.E-15));
#23255=DIRECTION('',(7.E-15,0.,1.));
#23256=DIRECTION('center_axis',(0.,1.,0.));
#23257=DIRECTION('ref_axis',(-1.,0.,7.E-15));
#23258=DIRECTION('',(7.E-15,0.,1.));
#23259=DIRECTION('center_axis',(-0.678851252797501,-0.734275817779166,4.75195876958251E-15));
#23260=DIRECTION('ref_axis',(7.E-15,1.94922383908984E-32,1.));
#23261=DIRECTION('',(-7.E-15,0.,-1.));
#23262=DIRECTION('',(-0.734275817779166,0.678851252797501,5.13993072445416E-15));
#23263=DIRECTION('',(7.E-15,0.,1.));
#23264=DIRECTION('',(7.E-15,0.,1.));
#23265=DIRECTION('',(-0.734275817779168,0.6788512527975,5.13993072445417E-15));
#23266=DIRECTION('center_axis',(-2.32761274233658E-16,-1.,1.6293289196356E-30));
#23267=DIRECTION('ref_axis',(7.E-15,-4.06124814761934E-47,1.));
#23268=DIRECTION('',(7.E-15,0.,1.));
#23269=DIRECTION('center_axis',(-0.678851252797501,-0.734275817779166,4.75195876958251E-15));
#23270=DIRECTION('ref_axis',(7.E-15,1.94922383908984E-32,1.));
#23271=DIRECTION('center_axis',(0.678851252797502,0.734275817779166,-4.75195876958251E-15));
#23272=DIRECTION('ref_axis',(0.734275817779166,-0.678851252797502,3.17141862916252E-30));
#23273=DIRECTION('center_axis',(-0.678851252797501,-0.734275817779166,4.75195876958251E-15));
#23274=DIRECTION('ref_axis',(7.E-15,1.94922383908984E-32,1.));
#23275=DIRECTION('center_axis',(0.678851252797499,0.734275817779168,-4.75195876958249E-15));
#23276=DIRECTION('ref_axis',(0.734275817779168,-0.678851252797499,-5.62097512108036E-30));
#23277=DIRECTION('center_axis',(-0.678851252797499,-0.734275817779168,4.75195876958249E-15));
#23278=DIRECTION('ref_axis',(-0.734275817779168,0.678851252797499,7.56831899889172E-30));
#23279=DIRECTION('center_axis',(0.678851252797499,0.734275817779168,-4.75195876958249E-15));
#23280=DIRECTION('ref_axis',(0.734275817779168,-0.678851252797499,-6.20021660737553E-30));
#23281=DIRECTION('',(-0.678851252797499,-0.734275817779168,4.75195876958249E-15));
#23282=DIRECTION('center_axis',(-0.6788512527975,-0.734275817779167,4.7519587695825E-15));
#23283=DIRECTION('ref_axis',(-0.734275817779167,0.6788512527975,2.81659329962846E-30));
#23284=DIRECTION('center_axis',(0.678851252797499,0.734275817779168,-4.75195876958249E-15));
#23285=DIRECTION('ref_axis',(0.734275817779168,-0.678851252797499,-5.62097512108036E-30));
#23286=DIRECTION('',(-0.6788512527975,-0.734275817779167,4.7519587695825E-15));
#23287=DIRECTION('center_axis',(7.E-15,0.,1.));
#23288=DIRECTION('ref_axis',(0.,-1.,0.));
#23289=DIRECTION('',(-0.734275817779168,0.6788512527975,5.13993072445417E-15));
#23290=DIRECTION('',(-0.734275817779168,0.6788512527975,5.13993072445417E-15));
#23291=DIRECTION('',(-0.6788512527975,-0.734275817779168,4.7519587695825E-15));
#23292=DIRECTION('',(-0.734275817779168,0.6788512527975,5.13993072445417E-15));
#23293=DIRECTION('',(-0.6788512527975,-0.734275817779168,4.7519587695825E-15));
#23294=DIRECTION('center_axis',(-0.734275817779167,0.6788512527975,5.13993072445417E-15));
#23295=DIRECTION('ref_axis',(7.E-15,9.31258724118286E-32,1.));
#23296=DIRECTION('',(-7.E-15,0.,-1.));
#23297=DIRECTION('',(-0.6788512527975,-0.734275817779168,4.7519587695825E-15));
#23298=DIRECTION('center_axis',(-7.E-15,0.,-1.));
#23299=DIRECTION('ref_axis',(-1.,0.,7.E-15));
#23300=DIRECTION('',(0.734275817779168,-0.6788512527975,-5.13993072445418E-15));
#23301=DIRECTION('',(0.734275817779168,-0.6788512527975,-5.13993072445417E-15));
#23302=DIRECTION('',(0.734275817779168,-0.6788512527975,-5.13993072445417E-15));
#23303=DIRECTION('',(-0.6788512527975,-0.734275817779168,4.7519587695825E-15));
#23304=DIRECTION('center_axis',(0.734275817779167,-0.6788512527975,-5.37545456543899E-15));
#23305=DIRECTION('ref_axis',(0.6788512527975,0.734275817779167,-4.7519587695825E-15));
#23306=DIRECTION('',(7.E-15,-3.46944695195362E-16,1.));
#23307=DIRECTION('',(7.E-15,-3.46944695195362E-16,1.));
#23308=DIRECTION('center_axis',(-0.6788512527975,-0.734275817779167,4.49720566979378E-15));
#23309=DIRECTION('ref_axis',(7.E-15,-3.46944695195361E-16,1.));
#23310=DIRECTION('center_axis',(-7.E-15,0.,-1.));
#23311=DIRECTION('ref_axis',(-1.,0.,7.E-15));
#23312=DIRECTION('',(0.774336703951835,0.632773789685546,-5.42035692766285E-15));
#23313=DIRECTION('',(0.734275817779166,-0.678851252797501,-5.13993072445416E-15));
#23314=DIRECTION('',(1.,3.96829847184794E-16,-7.E-15));
#23315=DIRECTION('center_axis',(-7.E-15,0.,-1.));
#23316=DIRECTION('ref_axis',(-1.,0.,7.E-15));
#23317=DIRECTION('',(0.,1.,0.));
#23318=DIRECTION('',(0.774336703951835,0.632773789685546,-5.42035692766285E-15));
#23319=DIRECTION('',(1.,3.96829847184794E-16,-7.E-15));
#23320=DIRECTION('',(0.734275817779166,-0.678851252797501,-5.13993072445416E-15));
#23321=DIRECTION('',(-1.,0.,7.E-15));
#23322=DIRECTION('',(-0.734275817779168,0.6788512527975,5.13993072445417E-15));
#23323=DIRECTION('center_axis',(0.6788512527975,0.734275817779167,-4.7519587695825E-15));
#23324=DIRECTION('ref_axis',(-7.E-15,5.87886466093466E-32,-1.));
#23325=DIRECTION('',(7.E-15,0.,1.));
#23326=DIRECTION('',(7.E-15,0.,1.));
#23327=DIRECTION('',(7.E-15,0.,1.));
#23328=DIRECTION('center_axis',(0.,1.,0.));
#23329=DIRECTION('ref_axis',(-1.,0.,7.E-15));
#23330=DIRECTION('',(7.E-15,0.,1.));
#23331=DIRECTION('',(7.E-15,0.,1.));
#23332=DIRECTION('',(7.E-15,0.,1.));
#23333=DIRECTION('center_axis',(-0.678851252797501,-0.734275817779166,4.75195876958251E-15));
#23334=DIRECTION('ref_axis',(7.E-15,1.94922383908984E-32,1.));
#23335=DIRECTION('',(7.E-15,0.,1.));
#23336=DIRECTION('',(7.E-15,0.,1.));
#23337=DIRECTION('',(7.E-15,0.,1.));
#23338=DIRECTION('center_axis',(3.96829847184794E-16,-1.,-2.77780893029356E-30));
#23339=DIRECTION('ref_axis',(1.,3.96829847184794E-16,-7.E-15));
#23340=DIRECTION('',(7.E-15,0.,1.));
#23341=DIRECTION('center_axis',(0.632773789685546,-0.774336703951836,-4.42941652779882E-15));
#23342=DIRECTION('ref_axis',(0.774336703951836,0.632773789685546,-5.42035692766285E-15));
#23343=DIRECTION('',(7.E-15,0.,1.));
#23344=DIRECTION('center_axis',(1.,0.,-7.E-15));
#23345=DIRECTION('ref_axis',(-7.E-15,0.,-1.));
#23346=DIRECTION('',(7.E-15,0.,1.));
#23347=DIRECTION('',(7.E-15,0.,1.));
#23348=DIRECTION('center_axis',(-0.6788512527975,-0.734275817779167,4.49720566979378E-15));
#23349=DIRECTION('ref_axis',(7.E-15,-3.46944695195361E-16,1.));
#23350=DIRECTION('center_axis',(3.96829847184794E-16,-1.,-2.77780893029356E-30));
#23351=DIRECTION('ref_axis',(1.,3.96829847184794E-16,-7.E-15));
#23352=DIRECTION('',(7.E-15,0.,1.));
#23353=DIRECTION('center_axis',(0.632773789685546,-0.774336703951836,-4.42941652779882E-15));
#23354=DIRECTION('ref_axis',(0.774336703951836,0.632773789685546,-5.42035692766285E-15));
#23355=DIRECTION('center_axis',(-9.98518434391482E-15,-1.,6.98962904074038E-29));
#23356=DIRECTION('ref_axis',(7.E-15,1.46992422332527E-45,1.));
#32971=CARTESIAN_POINT('',(0.,0.,0.));
#32972=CARTESIAN_POINT('Origin',(7.2492530515395,16.403587196458,205.));
#32973=CARTESIAN_POINT('',(8.18272201375405,19.4755763502051,205.));
#32974=CARTESIAN_POINT('Origin',(10.0893624969369,19.4755763502051,205.));
#32975=CARTESIAN_POINT('',(13.0097794346237,24.6967371281661,205.));
#32976=CARTESIAN_POINT('',(6.22126690664867,17.3539789503745,205.));
#32977=CARTESIAN_POINT('Origin',(14.0377655795145,23.7463453742496,205.));
#32978=CARTESIAN_POINT('Origin',(41.0259406693811,-14.8235704322271,205.));
#32979=CARTESIAN_POINT('',(41.0434612989213,-14.8397685706175,206.399796645178));
#32980=CARTESIAN_POINT('',(41.0434612989212,-14.8397685706175,203.600203354821));
#32981=CARTESIAN_POINT('',(41.0434612989212,-14.8397685706175,197.5));
#32982=CARTESIAN_POINT('',(39.9979545244903,-13.8731786783106,205.));
#32983=CARTESIAN_POINT('Origin',(41.0259406693811,-14.8235704322271,205.));
#32984=CARTESIAN_POINT('Origin',(41.0259406693811,-14.8235704322271,205.));
#32985=CARTESIAN_POINT('Origin',(41.0259406693811,-14.8235704322271,205.));
#32986=CARTESIAN_POINT('Origin',(41.0109651979399,-14.8397685706176,205.));
#32987=CARTESIAN_POINT('',(46.7864670524653,-6.53042050051894,205.));
#32988=CARTESIAN_POINT('',(39.9979545244903,-13.8731786783106,205.));
#32989=CARTESIAN_POINT('Origin',(47.8144531973562,-7.48081225443545,205.));
#32990=CARTESIAN_POINT('Origin',(-13.7460461167398,28.868260502022,212.5));
#32991=CARTESIAN_POINT('',(-81.5490276261588,28.8682605020227,201.188219076791));
#32992=CARTESIAN_POINT('',(-81.1900532671845,28.8682605020226,201.393647762688));
#32993=CARTESIAN_POINT('',(-81.5490276261588,28.8682605020227,201.188219076791));
#32994=CARTESIAN_POINT('',(-81.5490276261588,28.8682605020227,201.726680615253));
#32995=CARTESIAN_POINT('',(-81.5490276261588,28.8682605020227,201.726680615253));
#32996=CARTESIAN_POINT('',(-84.6900532671845,28.8682605020227,201.726680615253));
#32997=CARTESIAN_POINT('',(-84.6900532671845,28.8682605020227,201.726680615253));
#32998=CARTESIAN_POINT('',(-84.6900532671845,28.8682605020227,202.040783179355));
#32999=CARTESIAN_POINT('',(-84.6900532671845,28.8682605020227,202.040783179355));
#33000=CARTESIAN_POINT('',(-81.1900532671845,28.8682605020226,202.040783179355));
#33001=CARTESIAN_POINT('',(-81.1900532671845,28.8682605020226,202.040783179355));
#33002=CARTESIAN_POINT('',(-81.1900532671845,28.8682605020226,201.393647762688));
#33003=CARTESIAN_POINT('Origin',(-81.5490276261588,28.8682605020227,201.726680615253));
#33004=CARTESIAN_POINT('',(-81.5490276261588,29.0682605020227,201.726680615253));
#33005=CARTESIAN_POINT('',(-81.5490276261588,29.0682605020227,201.188219076791));
#33006=CARTESIAN_POINT('',(-81.5490276261588,29.0682605020227,201.726680615253));
#33007=CARTESIAN_POINT('',(-81.5490276261588,28.8682605020227,201.726680615253));
#33008=CARTESIAN_POINT('',(-81.5490276261588,28.8682605020227,201.188219076791));
#33009=CARTESIAN_POINT('Origin',(-84.6900532671845,28.8682605020227,201.726680615253));
#33010=CARTESIAN_POINT('',(-84.6900532671845,29.0682605020227,201.726680615253));
#33011=CARTESIAN_POINT('',(-84.6900532671845,29.0682605020227,201.726680615253));
#33012=CARTESIAN_POINT('',(-84.6900532671845,28.8682605020227,201.726680615253));
#33013=CARTESIAN_POINT('Origin',(-84.6900532671845,28.8682605020227,202.040783179355));
#33014=CARTESIAN_POINT('',(-84.6900532671845,29.0682605020227,202.040783179355));
#33015=CARTESIAN_POINT('',(-84.6900532671845,29.0682605020227,202.040783179355));
#33016=CARTESIAN_POINT('',(-84.6900532671845,28.8682605020227,202.040783179355));
#33017=CARTESIAN_POINT('Origin',(-81.1900532671845,28.8682605020226,202.040783179355));
#33018=CARTESIAN_POINT('',(-81.1900532671845,29.0682605020227,202.040783179355));
#33019=CARTESIAN_POINT('',(-81.1900532671845,29.0682605020227,202.040783179355));
#33020=CARTESIAN_POINT('',(-81.1900532671845,28.8682605020226,202.040783179355));
#33021=CARTESIAN_POINT('Origin',(-81.1900532671845,28.8682605020226,201.393647762688));
#33022=CARTESIAN_POINT('',(-81.1900532671845,29.0682605020227,201.393647762688));
#33023=CARTESIAN_POINT('',(-81.1900532671845,29.0682605020227,201.393647762688));
#33024=CARTESIAN_POINT('',(-81.1900532671845,28.8682605020226,201.393647762688));
#33025=CARTESIAN_POINT('Origin',(-81.5490276261588,28.8682605020227,201.188219076791));
#33026=CARTESIAN_POINT('',(-81.5490276261588,29.0682605020227,201.188219076791));
#33027=CARTESIAN_POINT('Origin',(-81.6887029333228,28.8682605020227,204.026105282754));
#33028=CARTESIAN_POINT('',(-81.4592840364153,28.8682605020227,204.601981096022));
#33029=CARTESIAN_POINT('',(-82.2669763441075,28.8682605020227,203.790783179355));
#33030=CARTESIAN_POINT('Ctrl Pts',(-81.4592840364153,28.8682605020227,204.601981096022));
#33031=CARTESIAN_POINT('Ctrl Pts',(-81.4599708546575,28.8682605020227,204.574603393385));
#33032=CARTESIAN_POINT('Ctrl Pts',(-81.4613196522816,28.8682605020227,204.520838105856));
#33033=CARTESIAN_POINT('Ctrl Pts',(-81.471536117869,28.8682605020227,204.442066315421));
#33034=CARTESIAN_POINT('Ctrl Pts',(-81.4870242844412,28.8682605020227,204.366402575227));
#33035=CARTESIAN_POINT('Ctrl Pts',(-81.5116228732431,28.8682605020227,204.294975855603));
#33036=CARTESIAN_POINT('Ctrl Pts',(-81.5406873285984,28.8682605020227,204.226239456265));
#33037=CARTESIAN_POINT('Ctrl Pts',(-81.5776105868505,28.8682605020227,204.161660790704));
#33038=CARTESIAN_POINT('Ctrl Pts',(-81.6205162333266,28.8682605020227,204.100167655303));
#33039=CARTESIAN_POINT('Ctrl Pts',(-81.6702670801791,28.8682605020227,204.042771493033));
#33040=CARTESIAN_POINT('Ctrl Pts',(-81.7261657529711,28.8682605020227,203.990350529552));
#33041=CARTESIAN_POINT('Ctrl Pts',(-81.7877699492256,28.8682605020227,203.943644208757));
#33042=CARTESIAN_POINT('Ctrl Pts',(-81.8546361678019,28.8682605020226,203.903103127741));
#33043=CARTESIAN_POINT('Ctrl Pts',(-81.9264899768362,28.8682605020227,203.867682009478));
#33044=CARTESIAN_POINT('Ctrl Pts',(-82.004046772439,28.8682605020227,203.838929655973));
#33045=CARTESIAN_POINT('Ctrl Pts',(-82.087013622034,28.8682605020227,203.816955559262));
#33046=CARTESIAN_POINT('Ctrl Pts',(-82.1750352431015,28.8682605020227,203.799568977673));
#33047=CARTESIAN_POINT('Ctrl Pts',(-82.2358202943267,28.8682605020227,203.793760419858));
#33048=CARTESIAN_POINT('Ctrl Pts',(-82.2669763441075,28.8682605020227,203.790783179355));
#33049=CARTESIAN_POINT('',(-82.1688192928255,28.8682605020227,205.361295999868));
#33050=CARTESIAN_POINT('Ctrl Pts',(-82.1688192928255,28.8682605020227,205.361295999868));
#33051=CARTESIAN_POINT('Ctrl Pts',(-82.1449378944147,28.8682605020227,205.360660257568));
#33052=CARTESIAN_POINT('Ctrl Pts',(-82.0978722440534,28.8682605020227,205.359407331577));
#33053=CARTESIAN_POINT('Ctrl Pts',(-82.0288664850348,28.8682605020227,205.348349634083));
#33054=CARTESIAN_POINT('Ctrl Pts',(-81.962301671219,28.8682605020227,205.331639127989));
#33055=CARTESIAN_POINT('Ctrl Pts',(-81.8979730521012,28.8682605020226,205.307693869941));
#33056=CARTESIAN_POINT('Ctrl Pts',(-81.836527400035,28.8682605020227,205.276087129855));
#33057=CARTESIAN_POINT('Ctrl Pts',(-81.7778899198314,28.8682605020226,205.237613749938));
#33058=CARTESIAN_POINT('Ctrl Pts',(-81.7212009546313,28.8682605020227,205.19322368652));
#33059=CARTESIAN_POINT('Ctrl Pts',(-81.6680476565732,28.8682605020226,205.141872417189));
#33060=CARTESIAN_POINT('Ctrl Pts',(-81.6193664510908,28.8682605020227,205.085460897382));
#33061=CARTESIAN_POINT('Ctrl Pts',(-81.5762423656764,28.8682605020226,205.025866647797));
#33062=CARTESIAN_POINT('Ctrl Pts',(-81.5402032548776,28.8682605020227,204.962816543537));
#33063=CARTESIAN_POINT('Ctrl Pts',(-81.5106597576971,28.8682605020226,204.896576421361));
#33064=CARTESIAN_POINT('Ctrl Pts',(-81.4874843765008,28.8682605020227,204.827330951953));
#33065=CARTESIAN_POINT('Ctrl Pts',(-81.4714257970777,28.8682605020227,204.754946206831));
#33066=CARTESIAN_POINT('Ctrl Pts',(-81.461343313131,28.8682605020227,204.679622190548));
#33067=CARTESIAN_POINT('Ctrl Pts',(-81.4599791412227,28.8682605020227,204.628188694857));
#33068=CARTESIAN_POINT('Ctrl Pts',(-81.4592840364153,28.8682605020227,204.601981096022));
#33069=CARTESIAN_POINT('',(-83.2415356389794,28.8682605020227,204.699437025509));
#33070=CARTESIAN_POINT('Ctrl Pts',(-83.2415356389794,28.8682605020227,204.699437025509));
#33071=CARTESIAN_POINT('Ctrl Pts',(-83.2070373324308,28.8682605020227,204.732484912317));
#33072=CARTESIAN_POINT('Ctrl Pts',(-83.1407731458266,28.8682605020227,204.795963139436));
#33073=CARTESIAN_POINT('Ctrl Pts',(-83.0440301856925,28.8682605020227,204.885745716245));
#33074=CARTESIAN_POINT('Ctrl Pts',(-82.9542806449404,28.8682605020227,204.966384704557));
#33075=CARTESIAN_POINT('Ctrl Pts',(-82.8716940964959,28.8682605020227,205.038402097329));
#33076=CARTESIAN_POINT('Ctrl Pts',(-82.7950625287004,28.8682605020227,205.100235602695));
#33077=CARTESIAN_POINT('Ctrl Pts',(-82.7268678251126,28.8682605020227,205.155107834643));
#33078=CARTESIAN_POINT('Ctrl Pts',(-82.6641133748048,28.8682605020227,205.199073425625));
#33079=CARTESIAN_POINT('Ctrl Pts',(-82.5913727608922,28.8682605020227,205.246788821312));
#33080=CARTESIAN_POINT('Ctrl Pts',(-82.5025604437182,28.8682605020227,205.293002802711));
#33081=CARTESIAN_POINT('Ctrl Pts',(-82.3940267544571,28.8682605020227,205.332715158751));
#33082=CARTESIAN_POINT('Ctrl Pts',(-82.2822995017811,28.8682605020226,205.3569300072));
#33083=CARTESIAN_POINT('Ctrl Pts',(-82.2067974647339,28.8682605020227,205.359834842706));
#33084=CARTESIAN_POINT('Ctrl Pts',(-82.1688192928255,28.8682605020227,205.361295999868));
#33085=CARTESIAN_POINT('',(-84.6900532671845,28.8682605020227,203.342065230637));
#33086=CARTESIAN_POINT('',(-84.6900532671845,28.8682605020227,203.342065230637));
#33087=CARTESIAN_POINT('',(-84.6900532671844,28.8682605020227,205.720270358842));
#33088=CARTESIAN_POINT('',(-84.6900532671844,28.8682605020227,205.720270358842));
#33089=CARTESIAN_POINT('',(-84.33107890821,28.8682605020227,205.720270358842));
#33090=CARTESIAN_POINT('',(-84.33107890821,28.8682605020227,205.720270358842));
#33091=CARTESIAN_POINT('',(-84.33107890821,28.8682605020227,204.091564429355));
#33092=CARTESIAN_POINT('',(-84.33107890821,28.8682605020227,204.091564429355));
#33093=CARTESIAN_POINT('',(-83.396483555646,28.8682605020227,204.96726555115));
#33094=CARTESIAN_POINT('',(-83.396483555646,28.8682605020227,204.96726555115));
#33095=CARTESIAN_POINT('',(-82.1407744210305,28.8682605020227,205.67539856397));
#33096=CARTESIAN_POINT('Ctrl Pts',(-82.1407744210305,28.8682605020227,205.67539856397));
#33097=CARTESIAN_POINT('Ctrl Pts',(-82.1895222346161,28.8682605020227,205.673705274502));
#33098=CARTESIAN_POINT('Ctrl Pts',(-82.2861624066765,28.8682605020227,205.670348410399));
#33099=CARTESIAN_POINT('Ctrl Pts',(-82.4281775770736,28.8682605020227,205.64163442389));
#33100=CARTESIAN_POINT('Ctrl Pts',(-82.5657698252851,28.8682605020227,205.596786428274));
#33101=CARTESIAN_POINT('Ctrl Pts',(-82.6765109016597,28.8682605020227,205.542793856741));
#33102=CARTESIAN_POINT('Ctrl Pts',(-82.7657359477164,28.8682605020227,205.488310702079));
#33103=CARTESIAN_POINT('Ctrl Pts',(-82.8392357134513,28.8682605020227,205.439262575613));
#33104=CARTESIAN_POINT('Ctrl Pts',(-82.9183543749108,28.8682605020227,205.381517084423));
#33105=CARTESIAN_POINT('Ctrl Pts',(-83.0034121639627,28.8682605020227,205.315567580555));
#33106=CARTESIAN_POINT('Ctrl Pts',(-83.0932951769942,28.8682605020227,205.240278319977));
#33107=CARTESIAN_POINT('Ctrl Pts',(-83.1898372690957,28.8682605020227,205.157605307559));
#33108=CARTESIAN_POINT('Ctrl Pts',(-83.2912533102384,28.8682605020227,205.065413484233));
#33109=CARTESIAN_POINT('Ctrl Pts',(-83.3605669592593,28.8682605020227,205.000764852468));
#33110=CARTESIAN_POINT('Ctrl Pts',(-83.396483555646,28.8682605020227,204.96726555115));
#33111=CARTESIAN_POINT('',(-81.1003096774409,28.8682605020226,204.618106897304));
#33112=CARTESIAN_POINT('Ctrl Pts',(-81.1003096774409,28.8682605020226,204.618106897304));
#33113=CARTESIAN_POINT('Ctrl Pts',(-81.1012008428613,28.8682605020226,204.656487672198));
#33114=CARTESIAN_POINT('Ctrl Pts',(-81.1029519510787,28.8682605020226,204.731904523843));
#33115=CARTESIAN_POINT('Ctrl Pts',(-81.1182161233739,28.8682605020226,204.841928331133));
#33116=CARTESIAN_POINT('Ctrl Pts',(-81.1416071069158,28.8682605020227,204.946917430261));
#33117=CARTESIAN_POINT('Ctrl Pts',(-81.1762688598019,28.8682605020226,205.045681980795));
#33118=CARTESIAN_POINT('Ctrl Pts',(-81.219761777561,28.8682605020227,205.139235584572));
#33119=CARTESIAN_POINT('Ctrl Pts',(-81.2738509190422,28.8682605020226,205.226419892733));
#33120=CARTESIAN_POINT('Ctrl Pts',(-81.3359769680758,28.8682605020227,205.309343112776));
#33121=CARTESIAN_POINT('Ctrl Pts',(-81.409257689452,28.8682605020227,205.383935517473));
#33122=CARTESIAN_POINT('Ctrl Pts',(-81.4874484042645,28.8682605020227,205.452457639886));
#33123=CARTESIAN_POINT('Ctrl Pts',(-81.5709554302159,28.8682605020226,205.51151956653));
#33124=CARTESIAN_POINT('Ctrl Pts',(-81.6573042663379,28.8682605020226,205.562384162401));
#33125=CARTESIAN_POINT('Ctrl Pts',(-81.7471694226447,28.8682605020227,205.604015245344));
#33126=CARTESIAN_POINT('Ctrl Pts',(-81.8408435437684,28.8682605020227,205.635573457601));
#33127=CARTESIAN_POINT('Ctrl Pts',(-81.937428543862,28.8682605020227,205.658955068432));
#33128=CARTESIAN_POINT('Ctrl Pts',(-82.0380390792887,28.8682605020227,205.672321260714));
#33129=CARTESIAN_POINT('Ctrl Pts',(-82.1061475940205,28.8682605020227,205.6743613625));
#33130=CARTESIAN_POINT('Ctrl Pts',(-82.1407744210305,28.8682605020227,205.67539856397));
#33131=CARTESIAN_POINT('',(-82.2669763441076,28.8682605020227,203.476680615253));
#33132=CARTESIAN_POINT('Ctrl Pts',(-82.2669763441076,28.8682605020227,203.476680615253));
#33133=CARTESIAN_POINT('Ctrl Pts',(-82.2253054563398,28.8682605020227,203.47872776826));
#33134=CARTESIAN_POINT('Ctrl Pts',(-82.1434649417649,28.8682605020227,203.482748322286));
#33135=CARTESIAN_POINT('Ctrl Pts',(-82.0241410353658,28.8682605020227,203.501576611548));
#33136=CARTESIAN_POINT('Ctrl Pts',(-81.9100862366409,28.8682605020227,203.528517488753));
#33137=CARTESIAN_POINT('Ctrl Pts',(-81.8022163226713,28.8682605020227,203.566608942768));
#33138=CARTESIAN_POINT('Ctrl Pts',(-81.6995775154409,28.8682605020226,203.613915220538));
#33139=CARTESIAN_POINT('Ctrl Pts',(-81.6025774997497,28.8682605020227,203.670645247919));
#33140=CARTESIAN_POINT('Ctrl Pts',(-81.511586311035,28.8682605020227,203.737839098432));
#33141=CARTESIAN_POINT('Ctrl Pts',(-81.4274474677396,28.8682605020226,203.814045832477));
#33142=CARTESIAN_POINT('Ctrl Pts',(-81.3502598969403,28.8682605020227,203.896814471532));
#33143=CARTESIAN_POINT('Ctrl Pts',(-81.2836046541341,28.8682605020227,203.986120411003));
#33144=CARTESIAN_POINT('Ctrl Pts',(-81.2272869827721,28.8682605020226,204.07996543829));
#33145=CARTESIAN_POINT('Ctrl Pts',(-81.1802057409483,28.8682605020227,204.178064837255));
#33146=CARTESIAN_POINT('Ctrl Pts',(-81.1448658950257,28.8682605020226,204.281525400815));
#33147=CARTESIAN_POINT('Ctrl Pts',(-81.1186442554211,28.8682605020226,204.389408258654));
#33148=CARTESIAN_POINT('Ctrl Pts',(-81.1028679096996,28.8682605020227,204.502187395063));
#33149=CARTESIAN_POINT('Ctrl Pts',(-81.1011721240953,28.8682605020226,204.57902741711));
#33150=CARTESIAN_POINT('Ctrl Pts',(-81.1003096774409,28.8682605020226,204.618106897304));
#33151=CARTESIAN_POINT('',(-82.2669763441075,28.8682605020227,203.790783179355));
#33152=CARTESIAN_POINT('Ctrl Pts',(-82.1688192928255,28.8682605020227,205.361295999868));
#33153=CARTESIAN_POINT('Ctrl Pts',(-82.1688192928255,29.1082605020227,205.361295999868));
#33154=CARTESIAN_POINT('Ctrl Pts',(-82.1449378944147,28.8682605020227,205.360660257568));
#33155=CARTESIAN_POINT('Ctrl Pts',(-82.1449378944147,29.1082605020227,205.360660257568));
#33156=CARTESIAN_POINT('Ctrl Pts',(-82.0978722440534,28.8682605020227,205.359407331577));
#33157=CARTESIAN_POINT('Ctrl Pts',(-82.0978722440534,29.1082605020227,205.359407331577));
#33158=CARTESIAN_POINT('Ctrl Pts',(-82.0288664850348,28.8682605020227,205.348349634083));
#33159=CARTESIAN_POINT('Ctrl Pts',(-82.0288664850348,29.1082605020227,205.348349634083));
#33160=CARTESIAN_POINT('Ctrl Pts',(-81.962301671219,28.8682605020227,205.331639127989));
#33161=CARTESIAN_POINT('Ctrl Pts',(-81.962301671219,29.1082605020227,205.331639127989));
#33162=CARTESIAN_POINT('Ctrl Pts',(-81.8979730521012,28.8682605020226,205.307693869941));
#33163=CARTESIAN_POINT('Ctrl Pts',(-81.8979730521012,29.1082605020226,205.307693869941));
#33164=CARTESIAN_POINT('Ctrl Pts',(-81.836527400035,28.8682605020227,205.276087129855));
#33165=CARTESIAN_POINT('Ctrl Pts',(-81.836527400035,29.1082605020227,205.276087129855));
#33166=CARTESIAN_POINT('Ctrl Pts',(-81.7778899198314,28.8682605020226,205.237613749938));
#33167=CARTESIAN_POINT('Ctrl Pts',(-81.7778899198314,29.1082605020226,205.237613749938));
#33168=CARTESIAN_POINT('Ctrl Pts',(-81.7212009546313,28.8682605020227,205.19322368652));
#33169=CARTESIAN_POINT('Ctrl Pts',(-81.7212009546313,29.1082605020227,205.19322368652));
#33170=CARTESIAN_POINT('Ctrl Pts',(-81.6680476565732,28.8682605020226,205.141872417189));
#33171=CARTESIAN_POINT('Ctrl Pts',(-81.6680476565732,29.1082605020226,205.141872417189));
#33172=CARTESIAN_POINT('Ctrl Pts',(-81.6193664510908,28.8682605020227,205.085460897382));
#33173=CARTESIAN_POINT('Ctrl Pts',(-81.6193664510908,29.1082605020227,205.085460897382));
#33174=CARTESIAN_POINT('Ctrl Pts',(-81.5762423656764,28.8682605020226,205.025866647797));
#33175=CARTESIAN_POINT('Ctrl Pts',(-81.5762423656764,29.1082605020226,205.025866647797));
#33176=CARTESIAN_POINT('Ctrl Pts',(-81.5402032548776,28.8682605020227,204.962816543537));
#33177=CARTESIAN_POINT('Ctrl Pts',(-81.5402032548776,29.1082605020227,204.962816543537));
#33178=CARTESIAN_POINT('Ctrl Pts',(-81.5106597576971,28.8682605020226,204.896576421361));
#33179=CARTESIAN_POINT('Ctrl Pts',(-81.5106597576971,29.1082605020226,204.896576421361));
#33180=CARTESIAN_POINT('Ctrl Pts',(-81.4874843765008,28.8682605020226,204.827330951953));
#33181=CARTESIAN_POINT('Ctrl Pts',(-81.4874843765008,29.1082605020226,204.827330951953));
#33182=CARTESIAN_POINT('Ctrl Pts',(-81.4714257970777,28.8682605020226,204.754946206831));
#33183=CARTESIAN_POINT('Ctrl Pts',(-81.4714257970777,29.1082605020226,204.754946206831));
#33184=CARTESIAN_POINT('Ctrl Pts',(-81.461343313131,28.8682605020226,204.679622190548));
#33185=CARTESIAN_POINT('Ctrl Pts',(-81.461343313131,29.1082605020226,204.679622190548));
#33186=CARTESIAN_POINT('Ctrl Pts',(-81.4599791412227,28.8682605020226,204.628188694857));
#33187=CARTESIAN_POINT('Ctrl Pts',(-81.4599791412227,29.1082605020226,204.628188694857));
#33188=CARTESIAN_POINT('Ctrl Pts',(-81.4592840364153,28.8682605020226,204.601981096022));
#33189=CARTESIAN_POINT('Ctrl Pts',(-81.4592840364153,29.1082605020226,204.601981096022));
#33190=CARTESIAN_POINT('',(-82.1688192928255,29.0682605020227,205.361295999868));
#33191=CARTESIAN_POINT('',(-81.4592840364153,29.0682605020227,204.601981096022));
#33192=CARTESIAN_POINT('Ctrl Pts',(-82.1688192928255,29.0682605020227,205.361295999868));
#33193=CARTESIAN_POINT('Ctrl Pts',(-82.1449378944147,29.0682605020227,205.360660257568));
#33194=CARTESIAN_POINT('Ctrl Pts',(-82.0978722440534,29.0682605020227,205.359407331577));
#33195=CARTESIAN_POINT('Ctrl Pts',(-82.0288664850348,29.0682605020227,205.348349634083));
#33196=CARTESIAN_POINT('Ctrl Pts',(-81.962301671219,29.0682605020227,205.331639127989));
#33197=CARTESIAN_POINT('Ctrl Pts',(-81.8979730521012,29.0682605020227,205.307693869941));
#33198=CARTESIAN_POINT('Ctrl Pts',(-81.836527400035,29.0682605020227,205.276087129855));
#33199=CARTESIAN_POINT('Ctrl Pts',(-81.7778899198314,29.0682605020227,205.237613749938));
#33200=CARTESIAN_POINT('Ctrl Pts',(-81.7212009546313,29.0682605020227,205.19322368652));
#33201=CARTESIAN_POINT('Ctrl Pts',(-81.6680476565732,29.0682605020227,205.141872417189));
#33202=CARTESIAN_POINT('Ctrl Pts',(-81.6193664510908,29.0682605020227,205.085460897382));
#33203=CARTESIAN_POINT('Ctrl Pts',(-81.5762423656764,29.0682605020227,205.025866647797));
#33204=CARTESIAN_POINT('Ctrl Pts',(-81.5402032548776,29.0682605020227,204.962816543537));
#33205=CARTESIAN_POINT('Ctrl Pts',(-81.5106597576971,29.0682605020226,204.896576421361));
#33206=CARTESIAN_POINT('Ctrl Pts',(-81.4874843765008,29.0682605020227,204.827330951953));
#33207=CARTESIAN_POINT('Ctrl Pts',(-81.4714257970777,29.0682605020227,204.754946206831));
#33208=CARTESIAN_POINT('Ctrl Pts',(-81.461343313131,29.0682605020227,204.679622190548));
#33209=CARTESIAN_POINT('Ctrl Pts',(-81.4599791412227,29.0682605020227,204.628188694857));
#33210=CARTESIAN_POINT('Ctrl Pts',(-81.4592840364153,29.0682605020227,204.601981096022));
#33211=CARTESIAN_POINT('',(-82.1688192928255,28.8682605020227,205.361295999868));
#33212=CARTESIAN_POINT('',(-81.4592840364153,28.8682605020227,204.601981096022));
#33213=CARTESIAN_POINT('Ctrl Pts',(-83.2415356389794,28.8682605020227,204.699437025509));
#33214=CARTESIAN_POINT('Ctrl Pts',(-83.2415356389794,29.1082605020227,204.699437025509));
#33215=CARTESIAN_POINT('Ctrl Pts',(-83.2070373324308,28.8682605020227,204.732484912317));
#33216=CARTESIAN_POINT('Ctrl Pts',(-83.2070373324308,29.1082605020227,204.732484912317));
#33217=CARTESIAN_POINT('Ctrl Pts',(-83.1407731458266,28.8682605020227,204.795963139436));
#33218=CARTESIAN_POINT('Ctrl Pts',(-83.1407731458266,29.1082605020227,204.795963139436));
#33219=CARTESIAN_POINT('Ctrl Pts',(-83.0440301856925,28.8682605020227,204.885745716245));
#33220=CARTESIAN_POINT('Ctrl Pts',(-83.0440301856925,29.1082605020227,204.885745716245));
#33221=CARTESIAN_POINT('Ctrl Pts',(-82.9542806449404,28.8682605020227,204.966384704557));
#33222=CARTESIAN_POINT('Ctrl Pts',(-82.9542806449404,29.1082605020227,204.966384704557));
#33223=CARTESIAN_POINT('Ctrl Pts',(-82.8716940964959,28.8682605020227,205.038402097329));
#33224=CARTESIAN_POINT('Ctrl Pts',(-82.8716940964959,29.1082605020227,205.038402097329));
#33225=CARTESIAN_POINT('Ctrl Pts',(-82.7950625287004,28.8682605020227,205.100235602695));
#33226=CARTESIAN_POINT('Ctrl Pts',(-82.7950625287004,29.1082605020227,205.100235602695));
#33227=CARTESIAN_POINT('Ctrl Pts',(-82.7268678251126,28.8682605020227,205.155107834643));
#33228=CARTESIAN_POINT('Ctrl Pts',(-82.7268678251126,29.1082605020227,205.155107834643));
#33229=CARTESIAN_POINT('Ctrl Pts',(-82.6641133748048,28.8682605020227,205.199073425625));
#33230=CARTESIAN_POINT('Ctrl Pts',(-82.6641133748048,29.1082605020227,205.199073425625));
#33231=CARTESIAN_POINT('Ctrl Pts',(-82.5913727608922,28.8682605020227,205.246788821312));
#33232=CARTESIAN_POINT('Ctrl Pts',(-82.5913727608922,29.1082605020227,205.246788821312));
#33233=CARTESIAN_POINT('Ctrl Pts',(-82.5025604437182,28.8682605020227,205.293002802711));
#33234=CARTESIAN_POINT('Ctrl Pts',(-82.5025604437182,29.1082605020227,205.293002802711));
#33235=CARTESIAN_POINT('Ctrl Pts',(-82.3940267544571,28.8682605020227,205.332715158751));
#33236=CARTESIAN_POINT('Ctrl Pts',(-82.3940267544571,29.1082605020227,205.332715158751));
#33237=CARTESIAN_POINT('Ctrl Pts',(-82.2822995017811,28.8682605020226,205.3569300072));
#33238=CARTESIAN_POINT('Ctrl Pts',(-82.2822995017811,29.1082605020226,205.3569300072));
#33239=CARTESIAN_POINT('Ctrl Pts',(-82.2067974647339,28.8682605020227,205.359834842706));
#33240=CARTESIAN_POINT('Ctrl Pts',(-82.2067974647339,29.1082605020227,205.359834842706));
#33241=CARTESIAN_POINT('Ctrl Pts',(-82.1688192928255,28.8682605020227,205.361295999868));
#33242=CARTESIAN_POINT('Ctrl Pts',(-82.1688192928255,29.1082605020227,205.361295999868));
#33243=CARTESIAN_POINT('',(-83.2415356389794,29.0682605020227,204.699437025509));
#33244=CARTESIAN_POINT('Ctrl Pts',(-83.2415356389794,29.0682605020227,204.699437025509));
#33245=CARTESIAN_POINT('Ctrl Pts',(-83.2070373324308,29.0682605020227,204.732484912317));
#33246=CARTESIAN_POINT('Ctrl Pts',(-83.1407731458266,29.0682605020227,204.795963139436));
#33247=CARTESIAN_POINT('Ctrl Pts',(-83.0440301856925,29.0682605020227,204.885745716245));
#33248=CARTESIAN_POINT('Ctrl Pts',(-82.9542806449404,29.0682605020227,204.966384704557));
#33249=CARTESIAN_POINT('Ctrl Pts',(-82.8716940964959,29.0682605020227,205.038402097329));
#33250=CARTESIAN_POINT('Ctrl Pts',(-82.7950625287004,29.0682605020227,205.100235602695));
#33251=CARTESIAN_POINT('Ctrl Pts',(-82.7268678251126,29.0682605020227,205.155107834643));
#33252=CARTESIAN_POINT('Ctrl Pts',(-82.6641133748048,29.0682605020227,205.199073425625));
#33253=CARTESIAN_POINT('Ctrl Pts',(-82.5913727608922,29.0682605020227,205.246788821312));
#33254=CARTESIAN_POINT('Ctrl Pts',(-82.5025604437182,29.0682605020227,205.293002802711));
#33255=CARTESIAN_POINT('Ctrl Pts',(-82.3940267544571,29.0682605020227,205.332715158751));
#33256=CARTESIAN_POINT('Ctrl Pts',(-82.2822995017811,29.0682605020227,205.3569300072));
#33257=CARTESIAN_POINT('Ctrl Pts',(-82.2067974647339,29.0682605020227,205.359834842706));
#33258=CARTESIAN_POINT('Ctrl Pts',(-82.1688192928255,29.0682605020227,205.361295999868));
#33259=CARTESIAN_POINT('',(-83.2415356389794,28.8682605020227,204.699437025509));
#33260=CARTESIAN_POINT('Origin',(-84.6900532671845,28.8682605020227,203.342065230637));
#33261=CARTESIAN_POINT('',(-84.6900532671845,29.0682605020227,203.342065230637));
#33262=CARTESIAN_POINT('',(-84.6900532671845,29.0682605020227,203.342065230637));
#33263=CARTESIAN_POINT('',(-84.6900532671845,28.8682605020227,203.342065230637));
#33264=CARTESIAN_POINT('Origin',(-84.6900532671844,28.8682605020227,205.720270358842));
#33265=CARTESIAN_POINT('',(-84.6900532671844,29.0682605020227,205.720270358842));
#33266=CARTESIAN_POINT('',(-84.6900532671844,29.0682605020227,205.720270358842));
#33267=CARTESIAN_POINT('',(-84.6900532671844,28.8682605020227,205.720270358842));
#33268=CARTESIAN_POINT('Origin',(-84.33107890821,28.8682605020227,205.720270358842));
#33269=CARTESIAN_POINT('',(-84.33107890821,29.0682605020227,205.720270358842));
#33270=CARTESIAN_POINT('',(-84.33107890821,29.0682605020227,205.720270358842));
#33271=CARTESIAN_POINT('',(-84.33107890821,28.8682605020227,205.720270358842));
#33272=CARTESIAN_POINT('Origin',(-84.33107890821,28.8682605020227,204.091564429355));
#33273=CARTESIAN_POINT('',(-84.33107890821,29.0682605020227,204.091564429355));
#33274=CARTESIAN_POINT('',(-84.33107890821,29.0682605020227,204.091564429355));
#33275=CARTESIAN_POINT('',(-84.33107890821,28.8682605020227,204.091564429355));
#33276=CARTESIAN_POINT('Origin',(-83.396483555646,28.8682605020227,204.96726555115));
#33277=CARTESIAN_POINT('',(-83.396483555646,29.0682605020227,204.96726555115));
#33278=CARTESIAN_POINT('',(-83.396483555646,29.0682605020227,204.96726555115));
#33279=CARTESIAN_POINT('',(-83.396483555646,28.8682605020227,204.96726555115));
#33280=CARTESIAN_POINT('Ctrl Pts',(-82.1407744210305,28.8682605020227,205.67539856397));
#33281=CARTESIAN_POINT('Ctrl Pts',(-82.1407744210305,29.1082605020227,205.67539856397));
#33282=CARTESIAN_POINT('Ctrl Pts',(-82.1895222346161,28.8682605020227,205.673705274502));
#33283=CARTESIAN_POINT('Ctrl Pts',(-82.1895222346161,29.1082605020227,205.673705274502));
#33284=CARTESIAN_POINT('Ctrl Pts',(-82.2861624066765,28.8682605020227,205.670348410399));
#33285=CARTESIAN_POINT('Ctrl Pts',(-82.2861624066765,29.1082605020227,205.670348410399));
#33286=CARTESIAN_POINT('Ctrl Pts',(-82.4281775770736,28.8682605020227,205.64163442389));
#33287=CARTESIAN_POINT('Ctrl Pts',(-82.4281775770736,29.1082605020227,205.64163442389));
#33288=CARTESIAN_POINT('Ctrl Pts',(-82.5657698252851,28.8682605020227,205.596786428274));
#33289=CARTESIAN_POINT('Ctrl Pts',(-82.5657698252851,29.1082605020227,205.596786428274));
#33290=CARTESIAN_POINT('Ctrl Pts',(-82.6765109016597,28.8682605020227,205.542793856741));
#33291=CARTESIAN_POINT('Ctrl Pts',(-82.6765109016597,29.1082605020227,205.542793856741));
#33292=CARTESIAN_POINT('Ctrl Pts',(-82.7657359477164,28.8682605020227,205.488310702079));
#33293=CARTESIAN_POINT('Ctrl Pts',(-82.7657359477164,29.1082605020227,205.488310702079));
#33294=CARTESIAN_POINT('Ctrl Pts',(-82.8392357134513,28.8682605020227,205.439262575613));
#33295=CARTESIAN_POINT('Ctrl Pts',(-82.8392357134513,29.1082605020227,205.439262575613));
#33296=CARTESIAN_POINT('Ctrl Pts',(-82.9183543749108,28.8682605020227,205.381517084423));
#33297=CARTESIAN_POINT('Ctrl Pts',(-82.9183543749108,29.1082605020227,205.381517084423));
#33298=CARTESIAN_POINT('Ctrl Pts',(-83.0034121639627,28.8682605020227,205.315567580555));
#33299=CARTESIAN_POINT('Ctrl Pts',(-83.0034121639627,29.1082605020227,205.315567580555));
#33300=CARTESIAN_POINT('Ctrl Pts',(-83.0932951769942,28.8682605020227,205.240278319977));
#33301=CARTESIAN_POINT('Ctrl Pts',(-83.0932951769942,29.1082605020227,205.240278319977));
#33302=CARTESIAN_POINT('Ctrl Pts',(-83.1898372690957,28.8682605020227,205.157605307559));
#33303=CARTESIAN_POINT('Ctrl Pts',(-83.1898372690957,29.1082605020227,205.157605307559));
#33304=CARTESIAN_POINT('Ctrl Pts',(-83.2912533102384,28.8682605020227,205.065413484233));
#33305=CARTESIAN_POINT('Ctrl Pts',(-83.2912533102384,29.1082605020227,205.065413484233));
#33306=CARTESIAN_POINT('Ctrl Pts',(-83.3605669592593,28.8682605020227,205.000764852468));
#33307=CARTESIAN_POINT('Ctrl Pts',(-83.3605669592593,29.1082605020227,205.000764852468));
#33308=CARTESIAN_POINT('Ctrl Pts',(-83.396483555646,28.8682605020227,204.96726555115));
#33309=CARTESIAN_POINT('Ctrl Pts',(-83.396483555646,29.1082605020227,204.96726555115));
#33310=CARTESIAN_POINT('',(-82.1407744210305,29.0682605020227,205.67539856397));
#33311=CARTESIAN_POINT('Ctrl Pts',(-82.1407744210305,29.0682605020227,205.67539856397));
#33312=CARTESIAN_POINT('Ctrl Pts',(-82.1895222346161,29.0682605020227,205.673705274502));
#33313=CARTESIAN_POINT('Ctrl Pts',(-82.2861624066765,29.0682605020227,205.670348410399));
#33314=CARTESIAN_POINT('Ctrl Pts',(-82.4281775770736,29.0682605020227,205.64163442389));
#33315=CARTESIAN_POINT('Ctrl Pts',(-82.5657698252851,29.0682605020227,205.596786428274));
#33316=CARTESIAN_POINT('Ctrl Pts',(-82.6765109016597,29.0682605020227,205.542793856741));
#33317=CARTESIAN_POINT('Ctrl Pts',(-82.7657359477164,29.0682605020227,205.488310702079));
#33318=CARTESIAN_POINT('Ctrl Pts',(-82.8392357134513,29.0682605020227,205.439262575613));
#33319=CARTESIAN_POINT('Ctrl Pts',(-82.9183543749108,29.0682605020227,205.381517084423));
#33320=CARTESIAN_POINT('Ctrl Pts',(-83.0034121639627,29.0682605020227,205.315567580555));
#33321=CARTESIAN_POINT('Ctrl Pts',(-83.0932951769942,29.0682605020227,205.240278319977));
#33322=CARTESIAN_POINT('Ctrl Pts',(-83.1898372690957,29.0682605020227,205.157605307559));
#33323=CARTESIAN_POINT('Ctrl Pts',(-83.2912533102384,29.0682605020227,205.065413484233));
#33324=CARTESIAN_POINT('Ctrl Pts',(-83.3605669592593,29.0682605020227,205.000764852468));
#33325=CARTESIAN_POINT('Ctrl Pts',(-83.396483555646,29.0682605020227,204.96726555115));
#33326=CARTESIAN_POINT('',(-82.1407744210305,28.8682605020227,205.67539856397));
#33327=CARTESIAN_POINT('Ctrl Pts',(-81.1003096774409,28.8682605020226,204.618106897304));
#33328=CARTESIAN_POINT('Ctrl Pts',(-81.1003096774409,29.1082605020227,204.618106897304));
#33329=CARTESIAN_POINT('Ctrl Pts',(-81.1012008428613,28.8682605020226,204.656487672198));
#33330=CARTESIAN_POINT('Ctrl Pts',(-81.1012008428613,29.1082605020227,204.656487672198));
#33331=CARTESIAN_POINT('Ctrl Pts',(-81.1029519510787,28.8682605020226,204.731904523843));
#33332=CARTESIAN_POINT('Ctrl Pts',(-81.1029519510787,29.1082605020227,204.731904523843));
#33333=CARTESIAN_POINT('Ctrl Pts',(-81.1182161233739,28.8682605020226,204.841928331133));
#33334=CARTESIAN_POINT('Ctrl Pts',(-81.1182161233739,29.1082605020227,204.841928331133));
#33335=CARTESIAN_POINT('Ctrl Pts',(-81.1416071069158,28.8682605020227,204.946917430261));
#33336=CARTESIAN_POINT('Ctrl Pts',(-81.1416071069158,29.1082605020227,204.946917430261));
#33337=CARTESIAN_POINT('Ctrl Pts',(-81.1762688598019,28.8682605020226,205.045681980795));
#33338=CARTESIAN_POINT('Ctrl Pts',(-81.1762688598019,29.1082605020227,205.045681980795));
#33339=CARTESIAN_POINT('Ctrl Pts',(-81.219761777561,28.8682605020227,205.139235584572));
#33340=CARTESIAN_POINT('Ctrl Pts',(-81.219761777561,29.1082605020227,205.139235584572));
#33341=CARTESIAN_POINT('Ctrl Pts',(-81.2738509190422,28.8682605020226,205.226419892733));
#33342=CARTESIAN_POINT('Ctrl Pts',(-81.2738509190422,29.1082605020227,205.226419892733));
#33343=CARTESIAN_POINT('Ctrl Pts',(-81.3359769680758,28.8682605020227,205.309343112776));
#33344=CARTESIAN_POINT('Ctrl Pts',(-81.3359769680758,29.1082605020227,205.309343112776));
#33345=CARTESIAN_POINT('Ctrl Pts',(-81.409257689452,28.8682605020227,205.383935517473));
#33346=CARTESIAN_POINT('Ctrl Pts',(-81.409257689452,29.1082605020227,205.383935517473));
#33347=CARTESIAN_POINT('Ctrl Pts',(-81.4874484042645,28.8682605020227,205.452457639886));
#33348=CARTESIAN_POINT('Ctrl Pts',(-81.4874484042645,29.1082605020227,205.452457639886));
#33349=CARTESIAN_POINT('Ctrl Pts',(-81.5709554302159,28.8682605020226,205.51151956653));
#33350=CARTESIAN_POINT('Ctrl Pts',(-81.5709554302159,29.1082605020227,205.51151956653));
#33351=CARTESIAN_POINT('Ctrl Pts',(-81.6573042663379,28.8682605020226,205.562384162401));
#33352=CARTESIAN_POINT('Ctrl Pts',(-81.6573042663379,29.1082605020227,205.562384162401));
#33353=CARTESIAN_POINT('Ctrl Pts',(-81.7471694226447,28.8682605020227,205.604015245344));
#33354=CARTESIAN_POINT('Ctrl Pts',(-81.7471694226447,29.1082605020227,205.604015245344));
#33355=CARTESIAN_POINT('Ctrl Pts',(-81.8408435437684,28.8682605020227,205.635573457601));
#33356=CARTESIAN_POINT('Ctrl Pts',(-81.8408435437684,29.1082605020227,205.635573457601));
#33357=CARTESIAN_POINT('Ctrl Pts',(-81.937428543862,28.8682605020227,205.658955068432));
#33358=CARTESIAN_POINT('Ctrl Pts',(-81.937428543862,29.1082605020227,205.658955068432));
#33359=CARTESIAN_POINT('Ctrl Pts',(-82.0380390792887,28.8682605020227,205.672321260714));
#33360=CARTESIAN_POINT('Ctrl Pts',(-82.0380390792887,29.1082605020227,205.672321260714));
#33361=CARTESIAN_POINT('Ctrl Pts',(-82.1061475940205,28.8682605020227,205.6743613625));
#33362=CARTESIAN_POINT('Ctrl Pts',(-82.1061475940205,29.1082605020227,205.6743613625));
#33363=CARTESIAN_POINT('Ctrl Pts',(-82.1407744210305,28.8682605020227,205.67539856397));
#33364=CARTESIAN_POINT('Ctrl Pts',(-82.1407744210305,29.1082605020227,205.67539856397));
#33365=CARTESIAN_POINT('',(-81.1003096774409,29.0682605020227,204.618106897304));
#33366=CARTESIAN_POINT('Ctrl Pts',(-81.1003096774409,29.0682605020227,204.618106897304));
#33367=CARTESIAN_POINT('Ctrl Pts',(-81.1012008428613,29.0682605020227,204.656487672198));
#33368=CARTESIAN_POINT('Ctrl Pts',(-81.1029519510787,29.0682605020227,204.731904523843));
#33369=CARTESIAN_POINT('Ctrl Pts',(-81.1182161233739,29.0682605020226,204.841928331133));
#33370=CARTESIAN_POINT('Ctrl Pts',(-81.1416071069158,29.0682605020227,204.946917430261));
#33371=CARTESIAN_POINT('Ctrl Pts',(-81.1762688598019,29.0682605020227,205.045681980795));
#33372=CARTESIAN_POINT('Ctrl Pts',(-81.219761777561,29.0682605020227,205.139235584572));
#33373=CARTESIAN_POINT('Ctrl Pts',(-81.2738509190422,29.0682605020226,205.226419892733));
#33374=CARTESIAN_POINT('Ctrl Pts',(-81.3359769680758,29.0682605020227,205.309343112776));
#33375=CARTESIAN_POINT('Ctrl Pts',(-81.409257689452,29.0682605020227,205.383935517473));
#33376=CARTESIAN_POINT('Ctrl Pts',(-81.4874484042645,29.0682605020227,205.452457639886));
#33377=CARTESIAN_POINT('Ctrl Pts',(-81.5709554302159,29.0682605020227,205.51151956653));
#33378=CARTESIAN_POINT('Ctrl Pts',(-81.6573042663379,29.0682605020226,205.562384162401));
#33379=CARTESIAN_POINT('Ctrl Pts',(-81.7471694226447,29.0682605020227,205.604015245344));
#33380=CARTESIAN_POINT('Ctrl Pts',(-81.8408435437684,29.0682605020227,205.635573457601));
#33381=CARTESIAN_POINT('Ctrl Pts',(-81.937428543862,29.0682605020227,205.658955068432));
#33382=CARTESIAN_POINT('Ctrl Pts',(-82.0380390792887,29.0682605020227,205.672321260714));
#33383=CARTESIAN_POINT('Ctrl Pts',(-82.1061475940205,29.0682605020227,205.6743613625));
#33384=CARTESIAN_POINT('Ctrl Pts',(-82.1407744210305,29.0682605020227,205.67539856397));
#33385=CARTESIAN_POINT('',(-81.1003096774409,28.8682605020226,204.618106897304));
#33386=CARTESIAN_POINT('Ctrl Pts',(-82.2669763441076,28.8682605020227,203.476680615253));
#33387=CARTESIAN_POINT('Ctrl Pts',(-82.2669763441076,29.1082605020227,203.476680615253));
#33388=CARTESIAN_POINT('Ctrl Pts',(-82.2253054563398,28.8682605020227,203.47872776826));
#33389=CARTESIAN_POINT('Ctrl Pts',(-82.2253054563398,29.1082605020227,203.47872776826));
#33390=CARTESIAN_POINT('Ctrl Pts',(-82.1434649417649,28.8682605020227,203.482748322286));
#33391=CARTESIAN_POINT('Ctrl Pts',(-82.1434649417649,29.1082605020227,203.482748322286));
#33392=CARTESIAN_POINT('Ctrl Pts',(-82.0241410353658,28.8682605020227,203.501576611548));
#33393=CARTESIAN_POINT('Ctrl Pts',(-82.0241410353658,29.1082605020227,203.501576611548));
#33394=CARTESIAN_POINT('Ctrl Pts',(-81.9100862366409,28.8682605020227,203.528517488753));
#33395=CARTESIAN_POINT('Ctrl Pts',(-81.9100862366409,29.1082605020227,203.528517488753));
#33396=CARTESIAN_POINT('Ctrl Pts',(-81.8022163226713,28.8682605020227,203.566608942768));
#33397=CARTESIAN_POINT('Ctrl Pts',(-81.8022163226713,29.1082605020227,203.566608942768));
#33398=CARTESIAN_POINT('Ctrl Pts',(-81.6995775154409,28.8682605020226,203.613915220538));
#33399=CARTESIAN_POINT('Ctrl Pts',(-81.6995775154409,29.1082605020226,203.613915220538));
#33400=CARTESIAN_POINT('Ctrl Pts',(-81.6025774997497,28.8682605020227,203.670645247919));
#33401=CARTESIAN_POINT('Ctrl Pts',(-81.6025774997497,29.1082605020227,203.670645247919));
#33402=CARTESIAN_POINT('Ctrl Pts',(-81.511586311035,28.8682605020227,203.737839098432));
#33403=CARTESIAN_POINT('Ctrl Pts',(-81.511586311035,29.1082605020227,203.737839098432));
#33404=CARTESIAN_POINT('Ctrl Pts',(-81.4274474677396,28.8682605020226,203.814045832477));
#33405=CARTESIAN_POINT('Ctrl Pts',(-81.4274474677396,29.1082605020226,203.814045832477));
#33406=CARTESIAN_POINT('Ctrl Pts',(-81.3502598969403,28.8682605020227,203.896814471532));
#33407=CARTESIAN_POINT('Ctrl Pts',(-81.3502598969403,29.1082605020227,203.896814471532));
#33408=CARTESIAN_POINT('Ctrl Pts',(-81.2836046541341,28.8682605020227,203.986120411003));
#33409=CARTESIAN_POINT('Ctrl Pts',(-81.2836046541341,29.1082605020227,203.986120411003));
#33410=CARTESIAN_POINT('Ctrl Pts',(-81.2272869827721,28.8682605020226,204.07996543829));
#33411=CARTESIAN_POINT('Ctrl Pts',(-81.2272869827721,29.1082605020226,204.07996543829));
#33412=CARTESIAN_POINT('Ctrl Pts',(-81.1802057409483,28.8682605020227,204.178064837255));
#33413=CARTESIAN_POINT('Ctrl Pts',(-81.1802057409483,29.1082605020227,204.178064837255));
#33414=CARTESIAN_POINT('Ctrl Pts',(-81.1448658950257,28.8682605020226,204.281525400815));
#33415=CARTESIAN_POINT('Ctrl Pts',(-81.1448658950257,29.1082605020226,204.281525400815));
#33416=CARTESIAN_POINT('Ctrl Pts',(-81.1186442554211,28.8682605020226,204.389408258654));
#33417=CARTESIAN_POINT('Ctrl Pts',(-81.1186442554211,29.1082605020226,204.389408258654));
#33418=CARTESIAN_POINT('Ctrl Pts',(-81.1028679096996,28.8682605020227,204.502187395063));
#33419=CARTESIAN_POINT('Ctrl Pts',(-81.1028679096996,29.1082605020227,204.502187395063));
#33420=CARTESIAN_POINT('Ctrl Pts',(-81.1011721240953,28.8682605020226,204.57902741711));
#33421=CARTESIAN_POINT('Ctrl Pts',(-81.1011721240953,29.1082605020226,204.57902741711));
#33422=CARTESIAN_POINT('Ctrl Pts',(-81.1003096774409,28.8682605020226,204.618106897304));
#33423=CARTESIAN_POINT('Ctrl Pts',(-81.1003096774409,29.1082605020226,204.618106897304));
#33424=CARTESIAN_POINT('',(-82.2669763441076,29.0682605020227,203.476680615253));
#33425=CARTESIAN_POINT('Ctrl Pts',(-82.2669763441076,29.0682605020227,203.476680615253));
#33426=CARTESIAN_POINT('Ctrl Pts',(-82.2253054563398,29.0682605020227,203.47872776826));
#33427=CARTESIAN_POINT('Ctrl Pts',(-82.1434649417649,29.0682605020227,203.482748322286));
#33428=CARTESIAN_POINT('Ctrl Pts',(-82.0241410353658,29.0682605020227,203.501576611548));
#33429=CARTESIAN_POINT('Ctrl Pts',(-81.9100862366409,29.0682605020227,203.528517488753));
#33430=CARTESIAN_POINT('Ctrl Pts',(-81.8022163226713,29.0682605020227,203.566608942768));
#33431=CARTESIAN_POINT('Ctrl Pts',(-81.6995775154409,29.0682605020227,203.613915220538));
#33432=CARTESIAN_POINT('Ctrl Pts',(-81.6025774997497,29.0682605020227,203.670645247919));
#33433=CARTESIAN_POINT('Ctrl Pts',(-81.511586311035,29.0682605020227,203.737839098432));
#33434=CARTESIAN_POINT('Ctrl Pts',(-81.4274474677396,29.0682605020226,203.814045832477));
#33435=CARTESIAN_POINT('Ctrl Pts',(-81.3502598969403,29.0682605020227,203.896814471532));
#33436=CARTESIAN_POINT('Ctrl Pts',(-81.2836046541341,29.0682605020227,203.986120411003));
#33437=CARTESIAN_POINT('Ctrl Pts',(-81.2272869827721,29.0682605020226,204.07996543829));
#33438=CARTESIAN_POINT('Ctrl Pts',(-81.1802057409483,29.0682605020227,204.178064837255));
#33439=CARTESIAN_POINT('Ctrl Pts',(-81.1448658950257,29.0682605020226,204.281525400815));
#33440=CARTESIAN_POINT('Ctrl Pts',(-81.1186442554211,29.0682605020227,204.389408258654));
#33441=CARTESIAN_POINT('Ctrl Pts',(-81.1028679096996,29.0682605020227,204.502187395063));
#33442=CARTESIAN_POINT('Ctrl Pts',(-81.1011721240953,29.0682605020227,204.57902741711));
#33443=CARTESIAN_POINT('Ctrl Pts',(-81.1003096774409,29.0682605020227,204.618106897304));
#33444=CARTESIAN_POINT('',(-82.2669763441076,28.8682605020227,203.476680615253));
#33445=CARTESIAN_POINT('Origin',(-82.2669763441075,28.8682605020227,203.790783179355));
#33446=CARTESIAN_POINT('',(-82.2669763441075,29.0682605020227,203.790783179355));
#33447=CARTESIAN_POINT('',(-82.2669763441075,29.0682605020227,203.790783179355));
#33448=CARTESIAN_POINT('',(-82.2669763441075,28.8682605020227,203.790783179355));
#33449=CARTESIAN_POINT('Ctrl Pts',(-81.4592840364153,28.8682605020227,204.601981096022));
#33450=CARTESIAN_POINT('Ctrl Pts',(-81.4592840364153,29.1082605020227,204.601981096022));
#33451=CARTESIAN_POINT('Ctrl Pts',(-81.4599708546575,28.8682605020227,204.574603393385));
#33452=CARTESIAN_POINT('Ctrl Pts',(-81.4599708546575,29.1082605020227,204.574603393385));
#33453=CARTESIAN_POINT('Ctrl Pts',(-81.4613196522816,28.8682605020227,204.520838105856));
#33454=CARTESIAN_POINT('Ctrl Pts',(-81.4613196522816,29.1082605020227,204.520838105856));
#33455=CARTESIAN_POINT('Ctrl Pts',(-81.471536117869,28.8682605020226,204.442066315421));
#33456=CARTESIAN_POINT('Ctrl Pts',(-81.471536117869,29.1082605020226,204.442066315421));
#33457=CARTESIAN_POINT('Ctrl Pts',(-81.4870242844412,28.8682605020226,204.366402575227));
#33458=CARTESIAN_POINT('Ctrl Pts',(-81.4870242844412,29.1082605020226,204.366402575227));
#33459=CARTESIAN_POINT('Ctrl Pts',(-81.5116228732431,28.8682605020227,204.294975855603));
#33460=CARTESIAN_POINT('Ctrl Pts',(-81.5116228732431,29.1082605020227,204.294975855603));
#33461=CARTESIAN_POINT('Ctrl Pts',(-81.5406873285984,28.8682605020226,204.226239456265));
#33462=CARTESIAN_POINT('Ctrl Pts',(-81.5406873285984,29.1082605020226,204.226239456265));
#33463=CARTESIAN_POINT('Ctrl Pts',(-81.5776105868505,28.8682605020226,204.161660790704));
#33464=CARTESIAN_POINT('Ctrl Pts',(-81.5776105868505,29.1082605020226,204.161660790704));
#33465=CARTESIAN_POINT('Ctrl Pts',(-81.6205162333266,28.8682605020227,204.100167655303));
#33466=CARTESIAN_POINT('Ctrl Pts',(-81.6205162333266,29.1082605020227,204.100167655303));
#33467=CARTESIAN_POINT('Ctrl Pts',(-81.6702670801791,28.8682605020227,204.042771493033));
#33468=CARTESIAN_POINT('Ctrl Pts',(-81.6702670801791,29.1082605020227,204.042771493033));
#33469=CARTESIAN_POINT('Ctrl Pts',(-81.7261657529711,28.8682605020226,203.990350529552));
#33470=CARTESIAN_POINT('Ctrl Pts',(-81.7261657529711,29.1082605020226,203.990350529552));
#33471=CARTESIAN_POINT('Ctrl Pts',(-81.7877699492256,28.8682605020227,203.943644208757));
#33472=CARTESIAN_POINT('Ctrl Pts',(-81.7877699492256,29.1082605020227,203.943644208757));
#33473=CARTESIAN_POINT('Ctrl Pts',(-81.8546361678019,28.8682605020226,203.903103127741));
#33474=CARTESIAN_POINT('Ctrl Pts',(-81.8546361678019,29.1082605020226,203.903103127741));
#33475=CARTESIAN_POINT('Ctrl Pts',(-81.9264899768362,28.8682605020227,203.867682009478));
#33476=CARTESIAN_POINT('Ctrl Pts',(-81.9264899768362,29.1082605020227,203.867682009478));
#33477=CARTESIAN_POINT('Ctrl Pts',(-82.004046772439,28.8682605020227,203.838929655973));
#33478=CARTESIAN_POINT('Ctrl Pts',(-82.004046772439,29.1082605020227,203.838929655973));
#33479=CARTESIAN_POINT('Ctrl Pts',(-82.087013622034,28.8682605020227,203.816955559262));
#33480=CARTESIAN_POINT('Ctrl Pts',(-82.087013622034,29.1082605020227,203.816955559262));
#33481=CARTESIAN_POINT('Ctrl Pts',(-82.1750352431015,28.8682605020227,203.799568977673));
#33482=CARTESIAN_POINT('Ctrl Pts',(-82.1750352431015,29.1082605020227,203.799568977673));
#33483=CARTESIAN_POINT('Ctrl Pts',(-82.2358202943267,28.8682605020227,203.793760419858));
#33484=CARTESIAN_POINT('Ctrl Pts',(-82.2358202943267,29.1082605020227,203.793760419858));
#33485=CARTESIAN_POINT('Ctrl Pts',(-82.2669763441075,28.8682605020227,203.790783179355));
#33486=CARTESIAN_POINT('Ctrl Pts',(-82.2669763441075,29.1082605020227,203.790783179355));
#33487=CARTESIAN_POINT('Ctrl Pts',(-81.4592840364153,29.0682605020227,204.601981096022));
#33488=CARTESIAN_POINT('Ctrl Pts',(-81.4599708546575,29.0682605020227,204.574603393385));
#33489=CARTESIAN_POINT('Ctrl Pts',(-81.4613196522816,29.0682605020227,204.520838105856));
#33490=CARTESIAN_POINT('Ctrl Pts',(-81.471536117869,29.0682605020227,204.442066315421));
#33491=CARTESIAN_POINT('Ctrl Pts',(-81.4870242844412,29.0682605020227,204.366402575227));
#33492=CARTESIAN_POINT('Ctrl Pts',(-81.5116228732431,29.0682605020227,204.294975855603));
#33493=CARTESIAN_POINT('Ctrl Pts',(-81.5406873285984,29.0682605020227,204.226239456265));
#33494=CARTESIAN_POINT('Ctrl Pts',(-81.5776105868505,29.0682605020227,204.161660790704));
#33495=CARTESIAN_POINT('Ctrl Pts',(-81.6205162333266,29.0682605020227,204.100167655303));
#33496=CARTESIAN_POINT('Ctrl Pts',(-81.6702670801791,29.0682605020227,204.042771493033));
#33497=CARTESIAN_POINT('Ctrl Pts',(-81.7261657529711,29.0682605020227,203.990350529552));
#33498=CARTESIAN_POINT('Ctrl Pts',(-81.7877699492256,29.0682605020227,203.943644208757));
#33499=CARTESIAN_POINT('Ctrl Pts',(-81.8546361678019,29.0682605020227,203.903103127741));
#33500=CARTESIAN_POINT('Ctrl Pts',(-81.9264899768362,29.0682605020227,203.867682009478));
#33501=CARTESIAN_POINT('Ctrl Pts',(-82.004046772439,29.0682605020227,203.838929655973));
#33502=CARTESIAN_POINT('Ctrl Pts',(-82.087013622034,29.0682605020227,203.816955559262));
#33503=CARTESIAN_POINT('Ctrl Pts',(-82.1750352431015,29.0682605020227,203.799568977673));
#33504=CARTESIAN_POINT('Ctrl Pts',(-82.2358202943267,29.0682605020227,203.793760419858));
#33505=CARTESIAN_POINT('Ctrl Pts',(-82.2669763441075,29.0682605020227,203.790783179355));
#33506=CARTESIAN_POINT('Origin',(18.6572199957115,29.0682605020217,207.25));
#33507=CARTESIAN_POINT('',(5.90651941603066,31.2638292831994,207.25));
#33508=CARTESIAN_POINT('',(-84.3160797324307,31.2638292832004,207.250000000001));
#33509=CARTESIAN_POINT('',(18.6572199957116,31.2638292831994,207.25));
#33510=CARTESIAN_POINT('',(8.28134461617001,29.0682605020218,207.25));
#33511=CARTESIAN_POINT('',(6.39609118240601,30.8112113446932,207.25));
#33512=CARTESIAN_POINT('',(-86.2573680265828,29.0682605020227,207.250000000001));
#33513=CARTESIAN_POINT('',(18.6572199957115,29.0682605020217,207.25));
#33514=CARTESIAN_POINT('',(-86.2573680265828,29.6774440008114,207.250000000001));
#33515=CARTESIAN_POINT('',(-86.2573680265828,29.0682605020227,207.250000000001));
#33516=CARTESIAN_POINT('',(-52.899264332329,56.9370761267468,207.25));
#33517=CARTESIAN_POINT('Origin',(18.6572199957116,31.2638292831994,207.25));
#33518=CARTESIAN_POINT('',(5.90651941603069,31.2638292831994,210.5));
#33519=CARTESIAN_POINT('',(-84.3160797324307,31.2638292832004,210.500000000001));
#33520=CARTESIAN_POINT('',(18.6572199957116,31.2638292831994,210.5));
#33521=CARTESIAN_POINT('',(5.9065194160306,31.2638292831994,197.5));
#33522=CARTESIAN_POINT('',(-84.3160797324308,31.2638292832004,197.500000000001));
#33523=CARTESIAN_POINT('Origin',(18.6572199957116,31.2638292831994,210.5));
#33524=CARTESIAN_POINT('',(4.59583969805239,32.4755763502034,210.5));
#33525=CARTESIAN_POINT('',(-82.8332429822645,32.4755763502043,210.5));
#33526=CARTESIAN_POINT('',(18.6572199957116,32.4755763502033,210.5));
#33527=CARTESIAN_POINT('',(6.39609118240604,30.8112113446932,210.5));
#33528=CARTESIAN_POINT('',(-52.899264332329,56.9370761267468,210.5));
#33529=CARTESIAN_POINT('Origin',(18.6572199957115,31.2755763502033,198.2));
#33530=CARTESIAN_POINT('',(5.8938132639902,31.2755763502035,198.2));
#33531=CARTESIAN_POINT('',(-84.3017046345787,31.2755763502044,198.200000000001));
#33532=CARTESIAN_POINT('',(18.6572199957115,31.2755763502033,198.2));
#33533=CARTESIAN_POINT('',(4.5958396980523,32.4755763502034,198.2));
#33534=CARTESIAN_POINT('',(6.39609118240595,30.8112113446932,198.2));
#33535=CARTESIAN_POINT('',(-82.8332429822646,32.4755763502043,198.200000000001));
#33536=CARTESIAN_POINT('',(18.6572199957115,32.4755763502033,198.2));
#33537=CARTESIAN_POINT('',(-52.8992643323291,56.9370761267468,198.2));
#33538=CARTESIAN_POINT('Origin',(18.6572199957115,31.2755763502033,199.2));
#33539=CARTESIAN_POINT('',(5.89381326399021,31.2755763502035,199.2));
#33540=CARTESIAN_POINT('',(-84.3017046345787,31.2755763502044,199.200000000001));
#33541=CARTESIAN_POINT('',(18.6572199957115,31.2755763502033,199.2));
#33542=CARTESIAN_POINT('',(5.8938132639902,31.2755763502035,197.5));
#33543=CARTESIAN_POINT('',(-84.3017046345787,31.2755763502044,197.500000000001));
#33544=CARTESIAN_POINT('Origin',(18.6572199957115,29.0682605020217,199.2));
#33545=CARTESIAN_POINT('',(-86.2573680265829,29.6774440008114,199.200000000001));
#33546=CARTESIAN_POINT('',(-86.2573680265829,29.0682605020227,199.200000000001));
#33547=CARTESIAN_POINT('',(-86.2573680265829,29.0682605020227,199.200000000001));
#33548=CARTESIAN_POINT('',(8.28134461616996,29.0682605020218,199.2));
#33549=CARTESIAN_POINT('',(18.6572199957115,29.0682605020217,199.2));
#33550=CARTESIAN_POINT('',(6.39609118240596,30.8112113446932,199.2));
#33551=CARTESIAN_POINT('',(-52.8992643323291,56.9370761267468,199.2));
#33552=CARTESIAN_POINT('Origin',(18.6572199957116,30.6104283104369,212.5));
#33553=CARTESIAN_POINT('',(6.61326707486714,30.6104283104371,211.828238018329));
#33554=CARTESIAN_POINT('',(-85.1156582925022,30.610428310438,211.82823801833));
#33555=CARTESIAN_POINT('',(18.6572199957116,30.6104283104369,211.828238018329));
#33556=CARTESIAN_POINT('',(6.61326707486715,30.6104283104371,212.5));
#33557=CARTESIAN_POINT('',(6.61326707486704,30.6104283104371,197.5));
#33558=CARTESIAN_POINT('',(-85.1156582925022,30.610428310438,212.500000000001));
#33559=CARTESIAN_POINT('',(-13.7460461167398,30.6104283104372,212.5));
#33560=CARTESIAN_POINT('',(-85.1156582925023,30.610428310438,197.500000000001));
#33561=CARTESIAN_POINT('Origin',(18.6572199957116,30.6104283104369,211.828238018329));
#33562=CARTESIAN_POINT('',(-86.2573680265828,29.6774440008114,211.82823801833));
#33563=CARTESIAN_POINT('',(-86.2573680265828,26.8977681671301,211.82823801833));
#33564=CARTESIAN_POINT('',(-86.2573680265828,30.610428310438,211.82823801833));
#33565=CARTESIAN_POINT('',(-78.2291940435082,19.4755763502051,211.82823801833));
#33566=CARTESIAN_POINT('',(-38.2529492465526,-17.4831838397085,211.82823801833));
#33567=CARTESIAN_POINT('',(18.6572199957114,19.4755763502041,211.828238018329));
#33568=CARTESIAN_POINT('',(18.6572199957114,19.4755763502041,211.828238018329));
#33569=CARTESIAN_POINT('',(6.39609118240605,30.8112113446932,211.828238018329));
#33570=CARTESIAN_POINT('',(-52.899264332329,56.9370761267468,211.82823801833));
#33571=CARTESIAN_POINT('Origin',(-38.2529492465528,-17.4831838397084,197.5));
#33572=CARTESIAN_POINT('',(-48.4539024103773,-8.05221843499776,205.));
#33573=CARTESIAN_POINT('Origin',(-47.2790611019306,-9.13838043947375,205.));
#33574=CARTESIAN_POINT('Origin',(-38.2529492465527,-17.4831838397085,197.5));
#33575=CARTESIAN_POINT('',(-80.7620383926607,21.8172366880922,205.));
#33576=CARTESIAN_POINT('Origin',(-79.587197084214,20.7310746836162,205.));
#33577=CARTESIAN_POINT('Origin',(-47.6184867283294,-9.50551834836335,205.));
#33578=CARTESIAN_POINT('',(-48.793328036776,-8.41935634388735,205.));
#33579=CARTESIAN_POINT('Origin',(-47.6184867283294,-9.50551834836335,205.));
#33580=CARTESIAN_POINT('',(-48.793328036776,-8.41935634388735,205.));
#33581=CARTESIAN_POINT('Origin',(-79.9266227106128,20.3639367747266,205.));
#33582=CARTESIAN_POINT('',(-81.1014640190594,21.4500987792026,205.));
#33583=CARTESIAN_POINT('Origin',(-79.9266227106128,20.3639367747266,205.));
#33584=CARTESIAN_POINT('',(-81.1014640190594,21.4500987792026,205.));
#33585=CARTESIAN_POINT('Origin',(-43.9471076394335,-12.8997746123508,209.));
#33586=CARTESIAN_POINT('',(-43.6076820130347,-12.5326367034613,209.));
#33587=CARTESIAN_POINT('',(-55.1735654967775,-1.83976857061746,209.));
#33588=CARTESIAN_POINT('',(-43.6076820130347,-12.5326367034613,209.));
#33589=CARTESIAN_POINT('',(-78.2291940435082,19.4755763502051,209.));
#33590=CARTESIAN_POINT('',(-43.6076820130347,-12.5326367034613,209.));
#33591=CARTESIAN_POINT('',(-83.2585761731098,24.1253309476037,209.));
#33592=CARTESIAN_POINT('',(-43.6076820130347,-12.5326367034613,209.));
#33593=CARTESIAN_POINT('',(-83.5980017995085,23.7581930387141,209.));
#33594=CARTESIAN_POINT('',(-83.5980017995085,23.7581930387141,209.));
#33595=CARTESIAN_POINT('',(-43.9471076394335,-12.8997746123508,209.));
#33596=CARTESIAN_POINT('',(-43.9471076394335,-12.8997746123508,209.));
#33597=CARTESIAN_POINT('',(-43.9471076394335,-12.8997746123508,209.));
#33598=CARTESIAN_POINT('Origin',(-43.9471076394335,-12.8997746123508,209.));
#33599=CARTESIAN_POINT('',(-43.6076820130348,-12.5326367034613,201.));
#33600=CARTESIAN_POINT('',(-43.6076820130347,-12.5326367034613,209.));
#33601=CARTESIAN_POINT('',(-43.9471076394335,-12.8997746123508,201.));
#33602=CARTESIAN_POINT('',(-43.9471076394335,-12.8997746123508,209.));
#33603=CARTESIAN_POINT('',(-43.9471076394335,-12.8997746123508,201.));
#33604=CARTESIAN_POINT('Origin',(-43.9471076394335,-12.8997746123508,201.));
#33605=CARTESIAN_POINT('',(-83.2585761731099,24.1253309476037,201.000000000001));
#33606=CARTESIAN_POINT('',(-78.2291940435083,19.4755763502051,201.));
#33607=CARTESIAN_POINT('',(-43.6076820130348,-12.5326367034613,201.));
#33608=CARTESIAN_POINT('',(-55.1735654967775,-1.8397685706175,201.));
#33609=CARTESIAN_POINT('',(-43.6076820130348,-12.5326367034613,201.));
#33610=CARTESIAN_POINT('',(-38.2529492465527,-17.4831838397084,201.));
#33611=CARTESIAN_POINT('',(-83.5980017995086,23.7581930387141,201.000000000001));
#33612=CARTESIAN_POINT('',(-43.9471076394335,-12.8997746123508,201.));
#33613=CARTESIAN_POINT('',(-83.5980017995086,23.7581930387141,201.000000000001));
#33614=CARTESIAN_POINT('Origin',(-83.5980017995085,23.7581930387141,209.));
#33615=CARTESIAN_POINT('',(-83.2585761731098,24.1253309476037,209.));
#33616=CARTESIAN_POINT('',(-83.5980017995085,23.7581930387141,209.));
#33617=CARTESIAN_POINT('Origin',(-38.5923748729513,-17.8503217485981,212.5));
#33618=CARTESIAN_POINT('Origin',(-38.2529492465526,-17.4831838397085,212.5));
#33619=CARTESIAN_POINT('',(-78.2291940435084,19.4755763502051,197.5));
#33620=CARTESIAN_POINT('',(-55.1735654967776,-1.8397685706175,197.5));
#33621=CARTESIAN_POINT('Origin',(-13.74604611674,9.02457653154,212.5));
#33622=CARTESIAN_POINT('',(-55.1735654967775,-1.8397685706175,212.5));
#33623=CARTESIAN_POINT('',(41.7128485424422,-1.8397685706175,212.5));
#33624=CARTESIAN_POINT('',(-13.74604611674,-1.8397685706175,212.5));
#33625=CARTESIAN_POINT('',(-41.1121851991166,-14.8397685706175,212.5));
#33626=CARTESIAN_POINT('',(-38.2529492465526,-17.4831838397084,212.5));
#33627=CARTESIAN_POINT('',(55.7742288401031,-14.8397685706175,212.499999999999));
#33628=CARTESIAN_POINT('',(-13.74604611674,-14.8397685706175,212.5));
#33629=CARTESIAN_POINT('',(6.39609118240605,30.8112113446932,212.5));
#33630=CARTESIAN_POINT('',(38.4592255574052,-7.8397685706175,212.5));
#33631=CARTESIAN_POINT('Origin',(40.4592255574052,-7.8397685706175,212.5));
#33632=CARTESIAN_POINT('',(-39.5407744425949,-7.8397685706175,212.5));
#33633=CARTESIAN_POINT('Origin',(-37.5407744425949,-7.8397685706175,212.5));
#33634=CARTESIAN_POINT('Origin',(-13.7460461167401,9.02457653154,197.5));
#33635=CARTESIAN_POINT('',(-55.1735654967776,-1.8397685706175,197.5));
#33636=CARTESIAN_POINT('',(41.7128485424421,-1.8397685706175,197.5));
#33637=CARTESIAN_POINT('',(-13.7460461167401,-1.8397685706175,197.5));
#33638=CARTESIAN_POINT('',(55.774228840103,-14.8397685706175,197.5));
#33639=CARTESIAN_POINT('',(6.39609118240595,30.8112113446932,197.5));
#33640=CARTESIAN_POINT('',(-41.1121851991167,-14.8397685706175,197.5));
#33641=CARTESIAN_POINT('',(-13.7460461167401,-14.8397685706175,197.5));
#33642=CARTESIAN_POINT('',(-38.2529492465528,-17.4831838397084,197.5));
#33643=CARTESIAN_POINT('',(38.4592255574051,-7.8397685706175,197.5));
#33644=CARTESIAN_POINT('Origin',(40.4592255574051,-7.8397685706175,197.5));
#33645=CARTESIAN_POINT('',(-39.540774442595,-7.8397685706175,197.5));
#33646=CARTESIAN_POINT('Origin',(-37.540774442595,-7.8397685706175,197.5));
#33647=CARTESIAN_POINT('Origin',(-38.2529492465528,-17.4831838397084,197.5));
#33648=CARTESIAN_POINT('',(-55.1735654967776,-1.8397685706175,197.5));
#33649=CARTESIAN_POINT('',(-41.1121851991167,-14.8397685706175,197.5));
#33650=CARTESIAN_POINT('',(-55.1735654967776,-1.8397685706175,197.5));
#33651=CARTESIAN_POINT('Origin',(-37.540774442595,-7.8397685706175,197.5));
#33652=CARTESIAN_POINT('',(-39.540774442595,-7.8397685706175,197.5));
#33653=CARTESIAN_POINT('Origin',(40.4592255574051,-7.8397685706175,197.5));
#33654=CARTESIAN_POINT('',(38.4592255574051,-7.8397685706175,197.5));
#33655=CARTESIAN_POINT('Origin',(-13.7460461167401,-14.8397685706175,197.5));
#33656=CARTESIAN_POINT('',(55.774228840103,-14.8397685706175,197.5));
#33657=CARTESIAN_POINT('Origin',(6.39609118240595,30.8112113446932,197.5));
#33658=CARTESIAN_POINT('',(50.7515564684729,-10.1962172656254,209.));
#33659=CARTESIAN_POINT('',(50.7515564684727,-10.1962172656254,199.));
#33660=CARTESIAN_POINT('',(50.7515564684728,-10.1962172656254,199.));
#33661=CARTESIAN_POINT('',(41.7128485424422,-1.8397685706175,209.));
#33662=CARTESIAN_POINT('',(50.7515564684729,-10.1962172656254,209.));
#33663=CARTESIAN_POINT('',(41.7128485424421,-1.8397685706175,197.5));
#33664=CARTESIAN_POINT('',(41.7128485424422,-1.83976857061742,199.));
#33665=CARTESIAN_POINT('',(41.7128485424421,-1.8397685706175,197.5));
#33666=CARTESIAN_POINT('',(50.7515564684728,-10.1962172656254,199.));
#33667=CARTESIAN_POINT('Origin',(-13.7460461167401,-1.8397685706175,197.5));
#33668=CARTESIAN_POINT('',(41.7128485424421,-1.8397685706175,197.5));
#33669=CARTESIAN_POINT('Origin',(6.39609118240595,30.8112113446932,197.5));
#33670=CARTESIAN_POINT('',(48.9892945058029,-8.56697425891133,205.));
#33671=CARTESIAN_POINT('Origin',(47.8144531973563,-7.48081225443535,205.));
#33672=CARTESIAN_POINT('Origin',(6.39609118240595,30.8112113446932,197.5));
#33673=CARTESIAN_POINT('',(15.2126068879612,22.6601833697736,205.));
#33674=CARTESIAN_POINT('Origin',(14.0377655795145,23.7463453742496,205.));
#33675=CARTESIAN_POINT('Origin',(48.0181085731954,-7.2605295091016,205.));
#33676=CARTESIAN_POINT('',(49.1929498816421,-8.3466915135776,205.));
#33677=CARTESIAN_POINT('Origin',(48.0181085731954,-7.2605295091016,205.));
#33678=CARTESIAN_POINT('',(49.1929498816421,-8.3466915135776,205.));
#33679=CARTESIAN_POINT('Origin',(14.2414209553537,23.9666281195834,205.));
#33680=CARTESIAN_POINT('',(15.4162622638004,22.8804661151074,205.));
#33681=CARTESIAN_POINT('Origin',(14.2414209553537,23.9666281195834,205.));
#33682=CARTESIAN_POINT('',(15.4162622638004,22.8804661151074,205.));
#33683=CARTESIAN_POINT('Origin',(50.9552118443121,-9.9759345202916,199.));
#33684=CARTESIAN_POINT('',(18.6572199957115,19.4755763502051,199.));
#33685=CARTESIAN_POINT('',(50.7515564684728,-10.1962172656254,199.));
#33686=CARTESIAN_POINT('',(9.63211067283946,27.8194528910347,199.));
#33687=CARTESIAN_POINT('',(50.7515564684728,-10.1962172656254,199.));
#33688=CARTESIAN_POINT('',(9.83576604867871,28.0397356363684,199.));
#33689=CARTESIAN_POINT('',(9.83576604867871,28.0397356363684,199.));
#33690=CARTESIAN_POINT('',(50.9552118443121,-9.9759345202916,199.));
#33691=CARTESIAN_POINT('',(50.9552118443121,-9.9759345202916,199.));
#33692=CARTESIAN_POINT('',(50.9552118443121,-9.9759345202916,199.));
#33693=CARTESIAN_POINT('Origin',(50.9552118443121,-9.9759345202916,199.));
#33694=CARTESIAN_POINT('',(50.9552118443122,-9.9759345202916,209.));
#33695=CARTESIAN_POINT('',(50.9552118443121,-9.9759345202916,199.));
#33696=CARTESIAN_POINT('',(50.9552118443122,-9.9759345202916,209.));
#33697=CARTESIAN_POINT('Origin',(50.9552118443122,-9.9759345202916,209.));
#33698=CARTESIAN_POINT('',(9.63211067283953,27.8194528910346,209.));
#33699=CARTESIAN_POINT('',(18.6572199957114,19.4755763502051,209.));
#33700=CARTESIAN_POINT('',(50.7515564684729,-10.1962172656254,209.));
#33701=CARTESIAN_POINT('',(50.7515564684729,-10.1962172656254,209.));
#33702=CARTESIAN_POINT('',(9.83576604867877,28.0397356363684,209.));
#33703=CARTESIAN_POINT('',(50.9552118443122,-9.9759345202916,209.));
#33704=CARTESIAN_POINT('',(9.83576604867877,28.0397356363684,209.));
#33705=CARTESIAN_POINT('Origin',(9.83576604867871,28.0397356363684,199.));
#33706=CARTESIAN_POINT('',(9.63211067283946,27.8194528910347,199.));
#33707=CARTESIAN_POINT('',(9.83576604867871,28.0397356363684,199.));
#33708=CARTESIAN_POINT('Origin',(6.5997465582453,31.031494090027,212.5));
#33709=CARTESIAN_POINT('Origin',(-13.74604611674,9.02457653154,212.5));
#33710=CARTESIAN_POINT('',(-82.8332429822645,32.4755763502051,212.5));
#33711=CARTESIAN_POINT('',(-52.899264332329,56.9370761267468,212.5));
#33712=CARTESIAN_POINT('',(4.59583969805065,32.4755763502051,212.5));
#33713=CARTESIAN_POINT('',(6.39609118240605,30.8112113446932,212.5));
#33714=CARTESIAN_POINT('',(-13.74604611674,32.4755763502051,212.5));
#33715=CARTESIAN_POINT('Origin',(-13.7460461167401,9.02457653154,197.5));
#33716=CARTESIAN_POINT('',(-86.2573680265831,26.8977681671302,197.500000000001));
#33717=CARTESIAN_POINT('',(-86.2573680265831,29.6774440008112,197.500000000001));
#33718=CARTESIAN_POINT('',(-86.2573680265831,9.02457653154,197.500000000001));
#33719=CARTESIAN_POINT('',(-82.8332429822646,32.4755763502051,197.500000000001));
#33720=CARTESIAN_POINT('',(-52.8992643323291,56.9370761267468,197.5));
#33721=CARTESIAN_POINT('',(4.59583969805055,32.4755763502051,197.5));
#33722=CARTESIAN_POINT('',(-13.7460461167401,32.4755763502051,197.5));
#33723=CARTESIAN_POINT('',(18.6572199957114,19.4755763502051,197.5));
#33724=CARTESIAN_POINT('',(6.39609118240595,30.8112113446932,197.5));
#33725=CARTESIAN_POINT('',(-78.2291940435083,19.4755763502051,197.5));
#33726=CARTESIAN_POINT('',(-13.7460461167401,19.4755763502051,197.5));
#33727=CARTESIAN_POINT('',(-38.2529492465527,-17.4831838397085,197.5));
#33728=CARTESIAN_POINT('Origin',(-38.2529492465527,-17.4831838397085,197.5));
#33729=CARTESIAN_POINT('',(-78.2291940435083,19.4755763502051,197.5));
#33730=CARTESIAN_POINT('',(-86.2573680265831,26.8977681671302,197.500000000001));
#33731=CARTESIAN_POINT('',(-78.2291940435083,19.4755763502051,197.5));
#33732=CARTESIAN_POINT('Origin',(-13.7460461167401,19.4755763502051,197.5));
#33733=CARTESIAN_POINT('',(18.6572199957114,19.4755763502051,197.5));
#33734=CARTESIAN_POINT('',(18.6572199957114,19.4755763502051,197.5));
#33735=CARTESIAN_POINT('',(18.6572199957114,19.4755763502051,197.5));
#33736=CARTESIAN_POINT('Origin',(6.39609118240595,30.8112113446932,197.5));
#33737=CARTESIAN_POINT('',(4.59583969805055,32.4755763502051,197.5));
#33738=CARTESIAN_POINT('',(8.28134461616995,29.0682605020218,197.5));
#33739=CARTESIAN_POINT('',(4.59583969805055,32.4755763502051,197.5));
#33740=CARTESIAN_POINT('Origin',(-13.7460461167401,32.4755763502051,197.5));
#33741=CARTESIAN_POINT('',(-82.8332429822646,32.4755763502051,197.500000000001));
#33742=CARTESIAN_POINT('Origin',(-52.8992643323291,56.9370761267468,197.5));
#33743=CARTESIAN_POINT('',(-86.2573680265831,29.6774440008112,197.500000000001));
#33744=CARTESIAN_POINT('Origin',(-86.2573680265831,9.02457653154,197.500000000001));
#33745=CARTESIAN_POINT('',(-86.2573680265829,29.0682605020227,199.200000000001));
#33746=CARTESIAN_POINT('',(-86.2573680265831,29.6774440008112,197.500000000001));
#33747=CARTESIAN_POINT('Origin',(6.39609118240605,30.8112113446933,212.5));
#33748=CARTESIAN_POINT('Origin',(-13.7460461167401,32.4755763502051,197.5));
#33749=CARTESIAN_POINT('',(-82.8332429822646,32.4755763502051,197.500000000001));
#33750=CARTESIAN_POINT('Origin',(-52.8992643323291,56.9370761267468,197.5));
#33751=CARTESIAN_POINT('Origin',(18.6572199957115,29.0682605020217,199.2));
#36653=UNCERTAINTY_MEASURE_WITH_UNIT(LENGTH_MEASURE(0.01),#36669,
'DISTANCE_ACCURACY_VALUE',
'Maximum model space distance between geometric entities at asserted c
onnectivities');
#36656=UNCERTAINTY_MEASURE_WITH_UNIT(LENGTH_MEASURE(0.01),#36669,
'DISTANCE_ACCURACY_VALUE',
'Maximum model space distance between geometric entities at asserted c
onnectivities');
#36665=(
GEOMETRIC_REPRESENTATION_CONTEXT(3)
GLOBAL_UNCERTAINTY_ASSIGNED_CONTEXT((#36653))
GLOBAL_UNIT_ASSIGNED_CONTEXT((#36669,#36671,#36672))
REPRESENTATION_CONTEXT('','3D')
);
#36668=(
GEOMETRIC_REPRESENTATION_CONTEXT(3)
GLOBAL_UNCERTAINTY_ASSIGNED_CONTEXT((#36656))
GLOBAL_UNIT_ASSIGNED_CONTEXT((#36669,#36671,#36672))
REPRESENTATION_CONTEXT('','3D')
);
#36669=(
LENGTH_UNIT()
NAMED_UNIT(*)
SI_UNIT(.MILLI.,.METRE.)
);
#36671=(
NAMED_UNIT(*)
PLANE_ANGLE_UNIT()
SI_UNIT($,.RADIAN.)
);
#36672=(
NAMED_UNIT(*)
SI_UNIT($,.STERADIAN.)
SOLID_ANGLE_UNIT()
);
#36681=SHAPE_DEFINITION_REPRESENTATION(#36692,#36713);
#36692=PRODUCT_DEFINITION_SHAPE('',$,#36725);
#36713=SHAPE_REPRESENTATION('',(#19085),#36665);
#36716=PRODUCT_DEFINITION_CONTEXT('part definition',#36751,'design');
#36725=PRODUCT_DEFINITION('Optical Tape Sensor Mount',
'Optical Tape Sensor Mount',#36736,#36716);
#36736=PRODUCT_DEFINITION_FORMATION('',$,#36761);
#36751=APPLICATION_CONTEXT(
'Core Data for Automotive Mechanical Design Process');
#36752=PRODUCT_CONTEXT('part definition',#36751,'mechanical');
#36761=PRODUCT('Optical Tape Sensor Mount','Optical Tape Sensor Mount',
$,(#36752));
#36769=PRESENTATION_STYLE_ASSIGNMENT((#36776));
#36776=SURFACE_STYLE_USAGE(.BOTH.,#36783);
#36783=SURFACE_SIDE_STYLE('',(#36790));
#36790=SURFACE_STYLE_FILL_AREA(#36797);
#36797=FILL_AREA_STYLE('Opaque(81,175,227)',(#36804));
#36804=FILL_AREA_STYLE_COLOUR('Opaque(81,175,227)',#36811);
#36811=COLOUR_RGB('Opaque(81,175,227)',0.317647058823529,0.686274509803922,
0.890196078431372);
ENDSEC;
END-ISO-10303-21;
